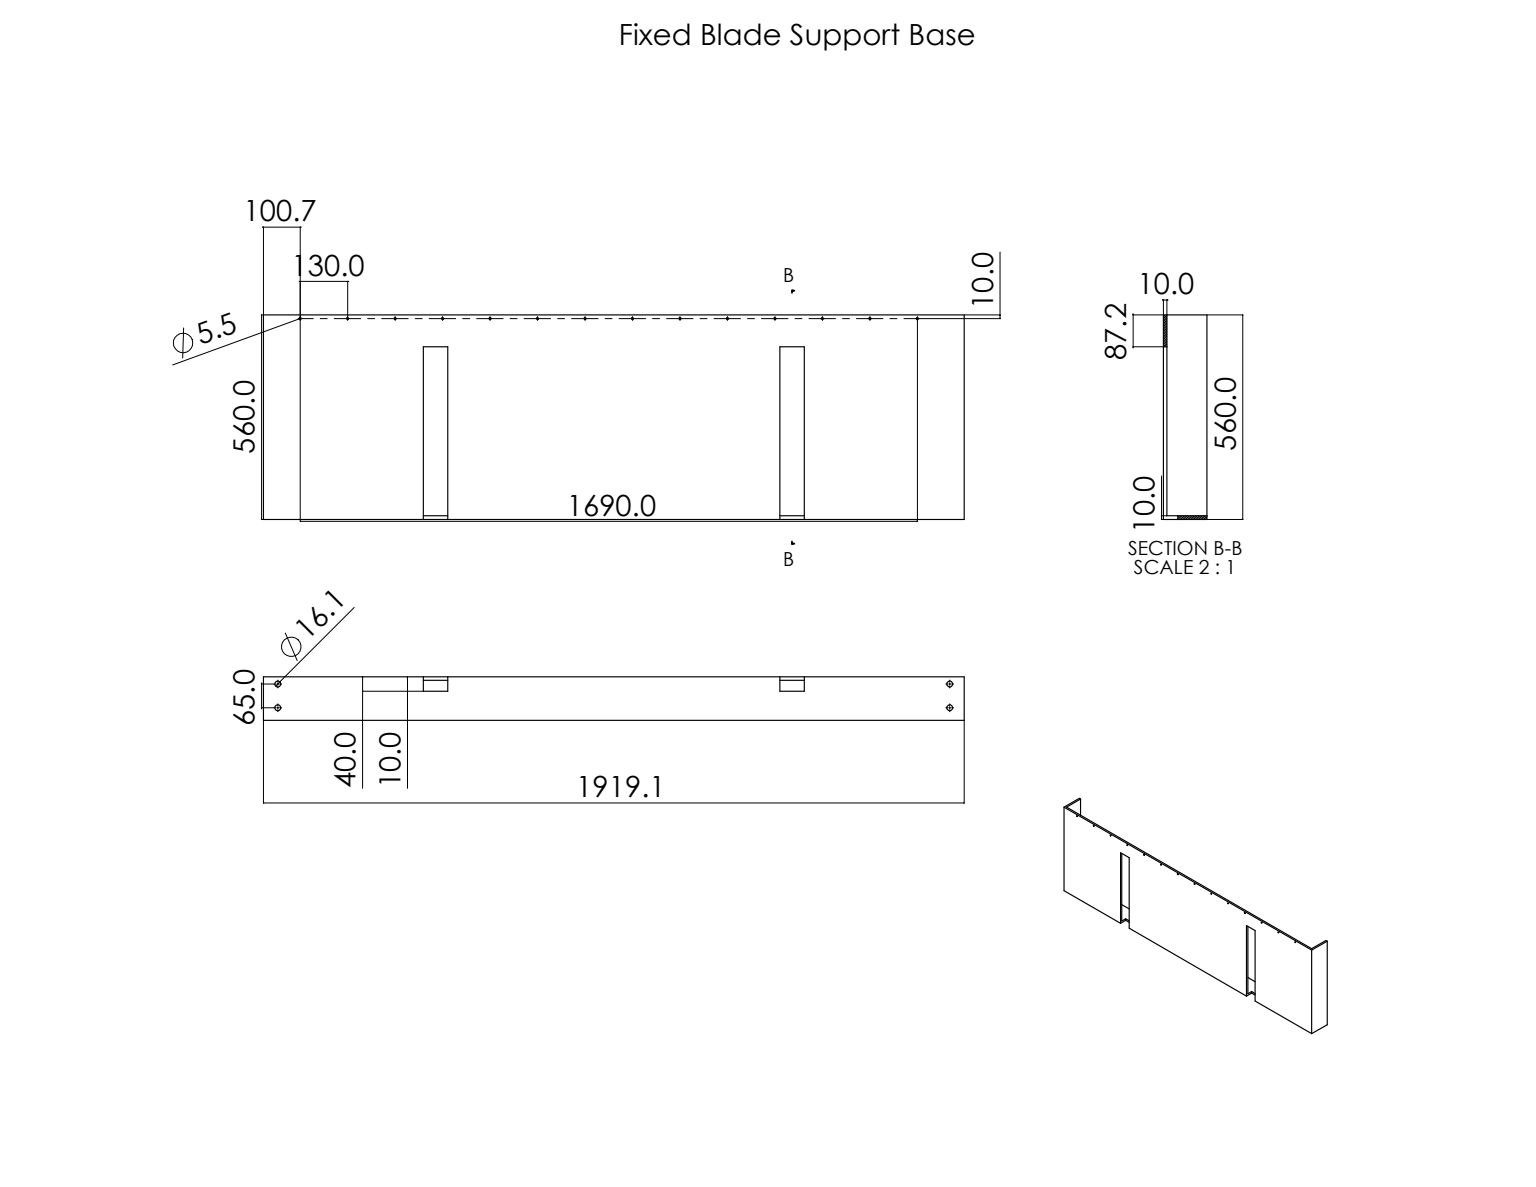
ISO-10303-21;
HEADER;
FILE_DESCRIPTION (('STEP AP214'),
    '1' );
FILE_NAME ('Fixed Blade Support Base.step',
    '2026-10-21T17:07:05',
    ( '' ),
    ( '' ),
    'SwSTEP 2.0',
    'SolidWorks 2025',
    '' );
FILE_SCHEMA (( 'AUTOMOTIVE_DESIGN' ));
ENDSEC;

DATA;
#38=ADVANCED_FACE ( 'NONE', ( #15558 ), #12093, .F. ) ;
#45=CARTESIAN_POINT ( 'NONE',  ( -454.7528517110260964, 240.0000000000001421, -122.7905160835438068 ) ) ;
#85=CARTESIAN_POINT ( 'NONE',  ( -949.5497976682736407, 240.0000000000002274, -2132.806278688367456 ) ) ;
#88=LINE ( 'NONE', #17428, #8305 ) ;
#95=DIRECTION ( 'NONE',  ( 1.000000000000000000, 0.000000000000000000, 0.000000000000000000 ) ) ;
#139=ORIENTED_EDGE ( 'NONE', *, *, #25849, .T. ) ;
#162=CARTESIAN_POINT ( 'NONE',  ( -208.8365100919714052, 260.0000000000001137, -197.2499999999928377 ) ) ;
#228=EDGE_LOOP ( 'NONE', ( #38649, #28007, #19169, #34955 ) ) ;
#282=VERTEX_POINT ( 'NONE', #6289 ) ;
#296=VERTEX_POINT ( 'NONE', #37011 ) ;
#303=CARTESIAN_POINT ( 'NONE',  ( -468.8365100919714337, 260.0000000000001705, -199.9999999999908766 ) ) ;
#305=ORIENTED_EDGE ( 'NONE', *, *, #27775, .T. ) ;
#308=DIRECTION ( 'NONE',  ( -1.880165489482579047E-16, -1.000000000000000000, -0.000000000000000000 ) ) ;
#338=VERTEX_POINT ( 'NONE', #40712 ) ;
#378=DIRECTION ( 'NONE',  ( -1.880165489482579047E-16, -1.000000000000000000, -0.000000000000000000 ) ) ;
#386=CIRCLE ( 'NONE', #29134, 2.749999999999919176 ) ;
#402=EDGE_CURVE ( 'NONE', #20839, #5125, #41180, .T. ) ;
#424=CARTESIAN_POINT ( 'NONE',  ( 454.7528517110262101, 239.9999999999999716, -122.7905160835442615 ) ) ;
#426=EDGE_CURVE ( 'NONE', #13538, #14856, #40502, .T. ) ;
#555=DIRECTION ( 'NONE',  ( -1.000000000000000000, 0.000000000000000000, 0.000000000000000000 ) ) ;
#590=ORIENTED_EDGE ( 'NONE', *, *, #29552, .T. ) ;
#593=VECTOR ( 'NONE', #7682, 1000.000000000000000 ) ;
#640=EDGE_CURVE ( 'NONE', #10075, #33702, #9985, .T. ) ;
#654=DIRECTION ( 'NONE',  ( -0.000000000000000000, 1.000000000000000000, -0.000000000000000000 ) ) ;
#709=ORIENTED_EDGE ( 'NONE', *, *, #5098, .T. ) ;
#718=ORIENTED_EDGE ( 'NONE', *, *, #22962, .T. ) ;
#728=EDGE_CURVE ( 'NONE', #13253, #15260, #21743, .T. ) ;
#739=CARTESIAN_POINT ( 'NONE',  ( 928.0249999999991815, 219.9999999999998863, 339.9999999999999432 ) ) ;
#767=ADVANCED_FACE ( 'NONE', ( #39786 ), #14838, .T. ) ;
#770=CARTESIAN_POINT ( 'NONE',  ( 919.9999999999993179, 154.9999999999998863, -360.0000000000000000 ) ) ;
#777=PLANE ( 'NONE',  #9882 ) ;
#791=VERTEX_POINT ( 'NONE', #739 ) ;
#796=CARTESIAN_POINT ( 'NONE',  ( -919.9999999999993179, 154.9999999999998863, 339.9999999999999432 ) ) ;
#804=ORIENTED_EDGE ( 'NONE', *, *, #1226, .T. ) ;
#824=CIRCLE ( 'NONE', #26615, 2.749999999999808153 ) ;
#853=( NAMED_UNIT ( * ) PLANE_ANGLE_UNIT ( ) SI_UNIT ( $, .RADIAN. ) );
#874=ORIENTED_EDGE ( 'NONE', *, *, #5250, .T. ) ;
#880=CARTESIAN_POINT ( 'NONE',  ( -728.8365100919714905, 260.0000000000001705, -197.2499999999891998 ) ) ;
#883=ORIENTED_EDGE ( 'NONE', *, *, #3255, .T. ) ;
#897=EDGE_LOOP ( 'NONE', ( #13761, #35388, #39807, #18362, #590, #6557 ) ) ;
#913=ADVANCED_FACE ( 'NONE', ( #39558 ), #7665, .T. ) ;
#925=CARTESIAN_POINT ( 'NONE',  ( 454.7528517110262101, 199.9999999999999432, -122.7905160835442615 ) ) ;
#928=VERTEX_POINT ( 'NONE', #4438 ) ;
#948=DIRECTION ( 'NONE',  ( -0.000000000000000000, 1.000000000000000000, -0.000000000000000000 ) ) ;
#955=EDGE_CURVE ( 'NONE', #16933, #23058, #18525, .T. ) ;
#977=ORIENTED_EDGE ( 'NONE', *, *, #34820, .T. ) ;
#990=CARTESIAN_POINT ( 'NONE',  ( -78.83651009197140525, 240.0000000000000853, -199.9999999999936051 ) ) ;
#999=CARTESIAN_POINT ( 'NONE',  ( -598.8365100919716042, 240.0000000000001705, -199.9999999999899671 ) ) ;
#1040=DIRECTION ( 'NONE',  ( -1.880165489482579047E-16, -1.000000000000000000, -0.000000000000000000 ) ) ;
#1042=ORIENTED_EDGE ( 'NONE', *, *, #30616, .F. ) ;
#1067=AXIS2_PLACEMENT_3D ( 'NONE', #33139, #27331, #40964 ) ;
#1084=AXIS2_PLACEMENT_3D ( 'NONE', #12147, #33380, #29263 ) ;
#1107=LINE ( 'NONE', #18453, #27055 ) ;
#1118=VECTOR ( 'NONE', #10969, 1000.000000000000000 ) ;
#1127=EDGE_LOOP ( 'NONE', ( #7257, #34123, #1263, #14595 ) ) ;
#1141=AXIS2_PLACEMENT_3D ( 'NONE', #10530, #3393, #38486 ) ;
#1148=AXIS2_PLACEMENT_3D ( 'NONE', #41013, #19989, #15837 ) ;
#1149=VECTOR ( 'NONE', #41633, 1000.000000000000000 ) ;
#1168=AXIS2_PLACEMENT_3D ( 'NONE', #303, #36103, #29173 ) ;
#1182=EDGE_CURVE ( 'NONE', #41190, #5430, #42343, .T. ) ;
#1199=EDGE_LOOP ( 'NONE', ( #16946, #35690 ) ) ;
#1226=EDGE_CURVE ( 'NONE', #32683, #45635, #5657, .T. ) ;
#1231=DIRECTION ( 'NONE',  ( 1.000000000000000000, 0.000000000000000000, 0.000000000000000000 ) ) ;
#1256=CARTESIAN_POINT ( 'NONE',  ( 919.9999999999993179, 219.9999999999998863, 339.9999999999999432 ) ) ;
#1263=ORIENTED_EDGE ( 'NONE', *, *, #19291, .T. ) ;
#1264=CARTESIAN_POINT ( 'NONE',  ( -208.8365100919714052, 240.0000000000001137, -199.9999999999926956 ) ) ;
#1270=AXIS2_PLACEMENT_3D ( 'NONE', #40692, #30517, #33770 ) ;
#1282=CARTESIAN_POINT ( 'NONE',  ( 521.6730038022808458, -9.808315785437627339E-14, 339.9999999999999432 ) ) ;
#1283=CARTESIAN_POINT ( 'NONE',  ( 454.7528517110261532, -8.550106180308601742E-14, 350.0000000000000000 ) ) ;
#1341=DIRECTION ( 'NONE',  ( -0.000000000000000000, 1.000000000000000000, -0.000000000000000000 ) ) ;
#1349=CARTESIAN_POINT ( 'NONE',  ( -521.6730038022808458, 230.0000000000001421, -122.7905160835438068 ) ) ;
#1382=VERTEX_POINT ( 'NONE', #27582 ) ;
#1385=CARTESIAN_POINT ( 'NONE',  ( -521.6730038022808458, 240.0000000000001705, -122.7905160835438068 ) ) ;
#1433=AXIS2_PLACEMENT_3D ( 'NONE', #27341, #16953, #45130 ) ;
#1438=CARTESIAN_POINT ( 'NONE',  ( 701.1634899080286232, 229.9999999999999147, -199.9999999999990337 ) ) ;
#1441=VERTEX_POINT ( 'NONE', #34968 ) ;
#1448=DIRECTION ( 'NONE',  ( -1.880165489482579047E-16, -1.000000000000000000, -0.000000000000000000 ) ) ;
#1468=UNCERTAINTY_MEASURE_WITH_UNIT (LENGTH_MEASURE( 1.000000000000000082E-05 ), #40729, 'distance_accuracy_value', 'NONE');
#1475=EDGE_CURVE ( 'NONE', #11526, #30518, #11359, .T. ) ;
#1533=EDGE_LOOP ( 'NONE', ( #21943, #37400, #33913, #3178 ) ) ;
#1581=EDGE_CURVE ( 'NONE', #44771, #12718, #29778, .T. ) ;
#1586=EDGE_LOOP ( 'NONE', ( #29834, #5171 ) ) ;
#1589=ADVANCED_FACE ( 'NONE', ( #18120 ), #7960, .F. ) ;
#1653=CARTESIAN_POINT ( 'NONE',  ( -858.8365100919713768, 240.0000000000002274, -197.2499999999882903 ) ) ;
#1658=CIRCLE ( 'NONE', #5350, 2.749999999999919176 ) ;
#1661=DIRECTION ( 'NONE',  ( 0.000000000000000000, 0.000000000000000000, 1.000000000000000000 ) ) ;
#1685=VERTEX_POINT ( 'NONE', #28739 ) ;
#1713=DIRECTION ( 'NONE',  ( 0.000000000000000000, 0.000000000000000000, 1.000000000000000000 ) ) ;
#1766=CYLINDRICAL_SURFACE ( 'NONE', #37801, 2.749999999999835687 ) ;
#1769=VERTEX_POINT ( 'NONE', #11404 ) ;
#1782=AXIS2_PLACEMENT_3D ( 'NONE', #9208, #19373, #33692 ) ;
#1802=EDGE_CURVE ( 'NONE', #5430, #41897, #11642, .T. ) ;
#1807=EDGE_CURVE ( 'NONE', #23028, #44488, #4925, .T. ) ;
#1818=AXIS2_PLACEMENT_3D ( 'NONE', #5730, #9193, #2253 ) ;
#1843=AXIS2_PLACEMENT_3D ( 'NONE', #23538, #17085, #9694 ) ;
#1872=EDGE_LOOP ( 'NONE', ( #17747, #14797 ) ) ;
#1891=CYLINDRICAL_SURFACE ( 'NONE', #26649, 2.749999999999863665 ) ;
#1902=FACE_BOUND ( 'NONE', #43260, .T. ) ;
#2009=PLANE ( 'NONE',  #5339 ) ;
#2099=VERTEX_POINT ( 'NONE', #40706 ) ;
#2160=EDGE_CURVE ( 'NONE', #33957, #338, #42375, .T. ) ;
#2235=CARTESIAN_POINT ( 'NONE',  ( 311.1634899080286232, 229.9999999999999716, -199.9999999999963336 ) ) ;
#2245=PRODUCT ( 'Fixed Blade Support Base', 'Fixed Blade Support Base', '', ( #30746 ) ) ;
#2253=DIRECTION ( 'NONE',  ( 1.000000000000000000, 0.000000000000000000, 0.000000000000000000 ) ) ;
#2263=DIRECTION ( 'NONE',  ( -1.880165489482579047E-16, -1.000000000000000000, -0.000000000000000000 ) ) ;
#2300=DIRECTION ( 'NONE',  ( 1.000000000000000000, 0.000000000000000000, 0.000000000000000000 ) ) ;
#2334=DIRECTION ( 'NONE',  ( 1.000000000000000000, -1.880165489482579047E-16, -0.000000000000000000 ) ) ;
#2362=CYLINDRICAL_SURFACE ( 'NONE', #32139, 2.749999999999863665 ) ;
#2393=DIRECTION ( 'NONE',  ( 0.000000000000000000, 0.000000000000000000, 1.000000000000000000 ) ) ;
#2412=CARTESIAN_POINT ( 'NONE',  ( -728.8365100919714905, 230.0000000000001705, -199.9999999999890861 ) ) ;
#2464=CARTESIAN_POINT ( 'NONE',  ( 571.1634899080285095, 259.9999999999999432, -197.2499999999982947 ) ) ;
#2466=ORIENTED_EDGE ( 'NONE', *, *, #29751, .T. ) ;
#2476=ORIENTED_EDGE ( 'NONE', *, *, #21855, .F. ) ;
#2503=AXIS2_PLACEMENT_3D ( 'NONE', #20702, #6847, #3401 ) ;
#2540=AXIS2_PLACEMENT_3D ( 'NONE', #20368, #24281, #24744 ) ;
#2545=EDGE_LOOP ( 'NONE', ( #19262, #7741, #30157, #11975 ) ) ;
#2557=AXIS2_PLACEMENT_3D ( 'NONE', #30153, #39499, #12154 ) ;
#2612=ORIENTED_EDGE ( 'NONE', *, *, #26636, .F. ) ;
#2616=DIRECTION ( 'NONE',  ( 0.000000000000000000, 0.000000000000000000, 1.000000000000000000 ) ) ;
#2632=ORIENTED_EDGE ( 'NONE', *, *, #41103, .T. ) ;
#2675=CARTESIAN_POINT ( 'NONE',  ( -454.7528517110260964, 240.0000000000001421, -122.7905160835438068 ) ) ;
#2710=ORIENTED_EDGE ( 'NONE', *, *, #30034, .T. ) ;
#2762=ORIENTED_EDGE ( 'NONE', *, *, #25210, .F. ) ;
#2775=CARTESIAN_POINT ( 'NONE',  ( -911.9749999999993406, 154.9999999999998863, -360.0000000000000000 ) ) ;
#2811=CARTESIAN_POINT ( 'NONE',  ( 51.16348990802859475, 230.0000000000000284, -197.2499999999946851 ) ) ;
#2837=DIRECTION ( 'NONE',  ( 0.000000000000000000, 0.000000000000000000, 1.000000000000000000 ) ) ;
#2846=DIRECTION ( 'NONE',  ( 0.000000000000000000, 0.000000000000000000, 1.000000000000000000 ) ) ;
#2882=DIRECTION ( 'NONE',  ( -0.000000000000000000, 1.000000000000000000, -0.000000000000000000 ) ) ;
#2940=CARTESIAN_POINT ( 'NONE',  ( 959.5497976682736407, 120.6654763175833693, -209.9999999999999716 ) ) ;
#2977=EDGE_LOOP ( 'NONE', ( #34128, #28219, #43060, #8539 ) ) ;
#3069=EDGE_LOOP ( 'NONE', ( #41787, #15073, #40615, #43520 ) ) ;
#3119=CIRCLE ( 'NONE', #40733, 2.749999999999863665 ) ;
#3178=ORIENTED_EDGE ( 'NONE', *, *, #9445, .F. ) ;
#3198=LINE ( 'NONE', #20529, #22575 ) ;
#3208=VECTOR ( 'NONE', #4412, 1000.000000000000000 ) ;
#3241=DIRECTION ( 'NONE',  ( 1.880165489482579047E-16, 1.000000000000000000, 0.000000000000000000 ) ) ;
#3255=EDGE_CURVE ( 'NONE', #5332, #39962, #34406, .T. ) ;
#3261=ORIENTED_EDGE ( 'NONE', *, *, #14766, .F. ) ;
#3301=FACE_OUTER_BOUND ( 'NONE', #15485, .T. ) ;
#3304=EDGE_LOOP ( 'NONE', ( #13111, #25405, #11101, #40410 ) ) ;
#3350=AXIS2_PLACEMENT_3D ( 'NONE', #35593, #3969, #7913 ) ;
#3392=CYLINDRICAL_SURFACE ( 'NONE', #42536, 2.749999999999835687 ) ;
#3393=DIRECTION ( 'NONE',  ( -0.000000000000000000, 1.000000000000000000, -0.000000000000000000 ) ) ;
#3397=DIRECTION ( 'NONE',  ( 1.000000000000000000, 0.000000000000000000, 0.000000000000000000 ) ) ;
#3401=DIRECTION ( 'NONE',  ( -1.000000000000000000, 0.000000000000000000, 0.000000000000000000 ) ) ;
#3427=VERTEX_POINT ( 'NONE', #29080 ) ;
#3447=EDGE_LOOP ( 'NONE', ( #7412, #17344 ) ) ;
#3452=DIRECTION ( 'NONE',  ( -0.000000000000000000, -0.000000000000000000, 1.000000000000000000 ) ) ;
#3455=VECTOR ( 'NONE', #31937, 1000.000000000000000 ) ;
#3458=AXIS2_PLACEMENT_3D ( 'NONE', #40138, #18451, #11058 ) ;
#3495=AXIS2_PLACEMENT_3D ( 'NONE', #13303, #23897, #38017 ) ;
#3503=ORIENTED_EDGE ( 'NONE', *, *, #13757, .T. ) ;
#3519=DIRECTION ( 'NONE',  ( 1.000000000000000000, 0.000000000000000000, 0.000000000000000000 ) ) ;
#3556=EDGE_LOOP ( 'NONE', ( #5524, #38328, #27108, #43854 ) ) ;
#3591=EDGE_CURVE ( 'NONE', #43844, #27381, #39729, .T. ) ;
#3630=DIRECTION ( 'NONE',  ( -0.000000000000000000, -0.000000000000000000, 1.000000000000000000 ) ) ;
#3650=ORIENTED_EDGE ( 'NONE', *, *, #36433, .F. ) ;
#3678=CARTESIAN_POINT ( 'NONE',  ( 521.6730038022808458, 199.9999999999999147, 350.0000000000000000 ) ) ;
#3695=FACE_BOUND ( 'NONE', #34718, .T. ) ;
#3710=DIRECTION ( 'NONE',  ( 1.000000000000000000, 0.000000000000000000, 0.000000000000000000 ) ) ;
#3770=ORIENTED_EDGE ( 'NONE', *, *, #22696, .F. ) ;
#3835=EDGE_LOOP ( 'NONE', ( #2476, #20852, #37122, #36881 ) ) ;
#3840=CYLINDRICAL_SURFACE ( 'NONE', #29331, 2.749999999999863665 ) ;
#3889=CARTESIAN_POINT ( 'NONE',  ( 949.5497976682736407, 229.9999999999998579, -210.0000000000000000 ) ) ;
#3943=CARTESIAN_POINT ( 'NONE',  ( 311.1634899080286232, 229.9999999999999716, -202.7499999999961915 ) ) ;
#3945=DIRECTION ( 'NONE',  ( -1.880165489482579047E-16, -1.000000000000000000, 0.000000000000000000 ) ) ;
#3957=DIRECTION ( 'NONE',  ( 1.000000000000000000, 0.000000000000000000, 0.000000000000000000 ) ) ;
#3969=DIRECTION ( 'NONE',  ( 4.147566128926363633E-16, 1.000000000000000000, -0.000000000000000000 ) ) ;
#4034=DIRECTION ( 'NONE',  ( -0.000000000000000000, -0.000000000000000000, 1.000000000000000000 ) ) ;
#4072=DIRECTION ( 'NONE',  ( -0.000000000000000000, 1.000000000000000000, -0.000000000000000000 ) ) ;
#4094=DIRECTION ( 'NONE',  ( 1.000000000000000000, -4.147566128926363633E-16, 0.000000000000000000 ) ) ;
#4099=AXIS2_PLACEMENT_3D ( 'NONE', #15118, #4034, #17897 ) ;
#4101=CARTESIAN_POINT ( 'NONE',  ( -598.8365100919716042, 230.0000000000001421, -199.9999999999899671 ) ) ;
#4111=EDGE_CURVE ( 'NONE', #1382, #39820, #21040, .T. ) ;
#4156=VECTOR ( 'NONE', #20629, 1000.000000000000000 ) ;
#4228=AXIS2_PLACEMENT_3D ( 'NONE', #19562, #44748, #44506 ) ;
#4250=DIRECTION ( 'NONE',  ( -0.000000000000000000, -0.000000000000000000, 1.000000000000000000 ) ) ;
#4263=DIRECTION ( 'NONE',  ( -1.880165489482579047E-16, -1.000000000000000000, -0.000000000000000000 ) ) ;
#4290=EDGE_LOOP ( 'NONE', ( #8058, #41150 ) ) ;
#4307=DIRECTION ( 'NONE',  ( -1.880165489482579047E-16, -1.000000000000000000, 0.000000000000000000 ) ) ;
#4314=CARTESIAN_POINT ( 'NONE',  ( 441.1634899080286232, 240.0000000000000000, -197.2499999999973852 ) ) ;
#4343=ORIENTED_EDGE ( 'NONE', *, *, #8870, .T. ) ;
#4355=FACE_BOUND ( 'NONE', #4290, .T. ) ;
#4357=CARTESIAN_POINT ( 'NONE',  ( -858.8365100919713768, 240.0000000000002274, -199.9999999999881481 ) ) ;
#4374=EDGE_CURVE ( 'NONE', #28460, #35455, #44677, .T. ) ;
#4408=ORIENTED_EDGE ( 'NONE', *, *, #39387, .F. ) ;
#4412=DIRECTION ( 'NONE',  ( 0.000000000000000000, 0.000000000000000000, 1.000000000000000000 ) ) ;
#4417=EDGE_CURVE ( 'NONE', #5332, #27330, #8529, .T. ) ;
#4438=CARTESIAN_POINT ( 'NONE',  ( 911.9749999999993406, 219.9999999999998863, 350.0000000000000000 ) ) ;
#4493=DIRECTION ( 'NONE',  ( -1.880165489482579047E-16, -1.000000000000000000, -0.000000000000000000 ) ) ;
#4501=DIRECTION ( 'NONE',  ( -0.000000000000000000, -0.000000000000000000, -1.000000000000000000 ) ) ;
#4503=ORIENTED_EDGE ( 'NONE', *, *, #34012, .T. ) ;
#4515=CARTESIAN_POINT ( 'NONE',  ( 51.16348990802859475, 230.0000000000000284, -199.9999999999945146 ) ) ;
#4523=CYLINDRICAL_SURFACE ( 'NONE', #21937, 2.749999999999835687 ) ;
#4528=PLANE ( 'NONE',  #30383 ) ;
#4587=CARTESIAN_POINT ( 'NONE',  ( -959.5497976682736407, 120.6654763175833693, 350.0000000000000000 ) ) ;
#4615=ORIENTED_EDGE ( 'NONE', *, *, #44639, .T. ) ;
#4617=EDGE_LOOP ( 'NONE', ( #37789, #37136, #11659, #3650 ) ) ;
#4645=EDGE_CURVE ( 'NONE', #13769, #7179, #33603, .T. ) ;
#4682=FACE_BOUND ( 'NONE', #31928, .T. ) ;
#4693=LINE ( 'NONE', #17881, #18176 ) ;
#4697=CIRCLE ( 'NONE', #30499, 2.749999999999863665 ) ;
#4724=ORIENTED_EDGE ( 'NONE', *, *, #38163, .F. ) ;
#4754=CARTESIAN_POINT ( 'NONE',  ( 51.16348990802859475, 240.0000000000000568, -199.9999999999945146 ) ) ;
#4780=AXIS2_PLACEMENT_3D ( 'NONE', #5364, #25726, #15110 ) ;
#4795=FACE_BOUND ( 'NONE', #34607, .T. ) ;
#4812=CIRCLE ( 'NONE', #1148, 8.024999999999948841 ) ;
#4841=CIRCLE ( 'NONE', #29926, 2.749999999999919176 ) ;
#4861=CIRCLE ( 'NONE', #30681, 8.024999999999948841 ) ;
#4901=ORIENTED_EDGE ( 'NONE', *, *, #1802, .F. ) ;
#4911=VECTOR ( 'NONE', #29518, 1000.000000000000000 ) ;
#4925=LINE ( 'NONE', #22028, #32023 ) ;
#4927=EDGE_CURVE ( 'NONE', #44845, #9329, #18884, .T. ) ;
#4933=CYLINDRICAL_SURFACE ( 'NONE', #4780, 2.749999999999863665 ) ;
#4939=AXIS2_PLACEMENT_3D ( 'NONE', #43926, #18779, #15992 ) ;
#4974=CIRCLE ( 'NONE', #12362, 8.024999999999948841 ) ;
#5098=EDGE_CURVE ( 'NONE', #12788, #16603, #29845, .T. ) ;
#5125=VERTEX_POINT ( 'NONE', #15541 ) ;
#5129=CIRCLE ( 'NONE', #1433, 2.749999999999835687 ) ;
#5139=EDGE_CURVE ( 'NONE', #34173, #10227, #7948, .T. ) ;
#5156=CARTESIAN_POINT ( 'NONE',  ( 959.5497976682736407, 239.9999999999998863, -2132.806278688367456 ) ) ;
#5160=DIRECTION ( 'NONE',  ( 1.000000000000000000, 0.000000000000000000, 0.000000000000000000 ) ) ;
#5171=ORIENTED_EDGE ( 'NONE', *, *, #43893, .T. ) ;
#5229=EDGE_LOOP ( 'NONE', ( #15133, #26425 ) ) ;
#5239=EDGE_CURVE ( 'NONE', #43290, #42970, #27072, .T. ) ;
#5249=CARTESIAN_POINT ( 'NONE',  ( 959.5497976682736407, 120.6654763175833693, -2132.806278688367456 ) ) ;
#5250=EDGE_CURVE ( 'NONE', #20839, #5289, #39638, .T. ) ;
#5289=VERTEX_POINT ( 'NONE', #30288 ) ;
#5332=VERTEX_POINT ( 'NONE', #40482 ) ;
#5339=AXIS2_PLACEMENT_3D ( 'NONE', #5930, #26716, #13330 ) ;
#5348=ORIENTED_EDGE ( 'NONE', *, *, #1226, .F. ) ;
#5350=AXIS2_PLACEMENT_3D ( 'NONE', #8388, #11398, #25483 ) ;
#5354=CARTESIAN_POINT ( 'NONE',  ( 831.1634899080286232, 229.9999999999998863, -197.2500000000000853 ) ) ;
#5364=CARTESIAN_POINT ( 'NONE',  ( 701.1634899080286232, 259.9999999999999432, -199.9999999999990337 ) ) ;
#5367=CIRCLE ( 'NONE', #26007, 2.749999999999863665 ) ;
#5371=DIRECTION ( 'NONE',  ( 0.000000000000000000, 0.000000000000000000, 1.000000000000000000 ) ) ;
#5384=CARTESIAN_POINT ( 'NONE',  ( 454.7528517110262101, 239.9999999999999716, -122.7905160835442615 ) ) ;
#5397=CARTESIAN_POINT ( 'NONE',  ( -919.9999999999993179, 154.9999999999998863, 350.0000000000000000 ) ) ;
#5414=DIRECTION ( 'NONE',  ( -1.880165489482579047E-16, -1.000000000000000000, -0.000000000000000000 ) ) ;
#5430=VERTEX_POINT ( 'NONE', #12737 ) ;
#5433=AXIS2_PLACEMENT_3D ( 'NONE', #22081, #32258, #21856 ) ;
#5446=ORIENTED_EDGE ( 'NONE', *, *, #32624, .F. ) ;
#5492=CARTESIAN_POINT ( 'NONE',  ( 311.1634899080286232, 240.0000000000000000, -202.7499999999961915 ) ) ;
#5496=ORIENTED_EDGE ( 'NONE', *, *, #20182, .F. ) ;
#5499=EDGE_CURVE ( 'NONE', #14856, #20856, #39484, .T. ) ;
#5503=EDGE_LOOP ( 'NONE', ( #40837, #6028 ) ) ;
#5506=VECTOR ( 'NONE', #5595, 1000.000000000000000 ) ;
#5522=VECTOR ( 'NONE', #4307, 1000.000000000000000 ) ;
#5524=ORIENTED_EDGE ( 'NONE', *, *, #32500, .T. ) ;
#5541=EDGE_CURVE ( 'NONE', #6874, #9331, #11602, .T. ) ;
#5585=ORIENTED_EDGE ( 'NONE', *, *, #17111, .F. ) ;
#5591=DIRECTION ( 'NONE',  ( -0.000000000000000000, 1.000000000000000000, -0.000000000000000000 ) ) ;
#5595=DIRECTION ( 'NONE',  ( 1.000000000000000000, -1.880165489482579047E-16, -0.000000000000000000 ) ) ;
#5626=ORIENTED_EDGE ( 'NONE', *, *, #14615, .F. ) ;
#5635=FACE_BOUND ( 'NONE', #29931, .T. ) ;
#5638=CARTESIAN_POINT ( 'NONE',  ( -949.5497976682736407, 120.6654763175833693, -2132.806278688367456 ) ) ;
#5657=LINE ( 'NONE', #34278, #45285 ) ;
#5679=DIRECTION ( 'NONE',  ( -0.000000000000000000, 1.000000000000000000, -0.000000000000000000 ) ) ;
#5694=ORIENTED_EDGE ( 'NONE', *, *, #44442, .T. ) ;
#5710=LINE ( 'NONE', #23474, #20423 ) ;
#5717=DIRECTION ( 'NONE',  ( 1.000000000000000000, 0.000000000000000000, 0.000000000000000000 ) ) ;
#5730=CARTESIAN_POINT ( 'NONE',  ( 919.9999999999993179, 219.9999999999998863, -360.0000000000000000 ) ) ;
#5760=LINE ( 'NONE', #33929, #19426 ) ;
#5802=ORIENTED_EDGE ( 'NONE', *, *, #33989, .F. ) ;
#5810=VERTEX_POINT ( 'NONE', #1349 ) ;
#5814=ADVANCED_FACE ( 'NONE', ( #19974 ), #36448, .T. ) ;
#5820=LINE ( 'NONE', #16902, #44029 ) ;
#5848=VERTEX_POINT ( 'NONE', #15229 ) ;
#5869=FACE_OUTER_BOUND ( 'NONE', #22229, .T. ) ;
#5870=ORIENTED_EDGE ( 'NONE', *, *, #15575, .F. ) ;
#5906=CARTESIAN_POINT ( 'NONE',  ( -911.9749999999993406, 219.9999999999998863, 339.9999999999999432 ) ) ;
#5930=CARTESIAN_POINT ( 'NONE',  ( 454.7528517110262101, 199.9999999999999432, -122.7905160835442615 ) ) ;
#5955=VERTEX_POINT ( 'NONE', #4587 ) ;
#5978=VERTEX_POINT ( 'NONE', #9357 ) ;
#6013=AXIS2_PLACEMENT_3D ( 'NONE', #18296, #15281, #3957 ) ;
#6028=ORIENTED_EDGE ( 'NONE', *, *, #5250, .F. ) ;
#6075=DIRECTION ( 'NONE',  ( 1.000000000000000000, 0.000000000000000000, 0.000000000000000000 ) ) ;
#6093=ORIENTED_EDGE ( 'NONE', *, *, #29552, .F. ) ;
#6158=DIRECTION ( 'NONE',  ( 1.000000000000000000, 0.000000000000000000, 0.000000000000000000 ) ) ;
#6177=FACE_BOUND ( 'NONE', #14391, .T. ) ;
#6189=EDGE_LOOP ( 'NONE', ( #30273, #41536 ) ) ;
#6220=DIRECTION ( 'NONE',  ( -0.000000000000000000, 1.000000000000000000, -0.000000000000000000 ) ) ;
#6225=CARTESIAN_POINT ( 'NONE',  ( 959.5497976682736407, 120.6654763175833693, -209.9999999999999716 ) ) ;
#6264=CARTESIAN_POINT ( 'NONE',  ( -911.9749999999993406, 154.9999999999998863, 350.0000000000000000 ) ) ;
#6289=CARTESIAN_POINT ( 'NONE',  ( 928.0249999999991815, 219.9999999999998863, 350.0000000000000000 ) ) ;
#6316=ORIENTED_EDGE ( 'NONE', *, *, #42173, .T. ) ;
#6322=DIRECTION ( 'NONE',  ( -0.000000000000000000, 1.000000000000000000, -0.000000000000000000 ) ) ;
#6330=CARTESIAN_POINT ( 'NONE',  ( 8.295132257852724189E-14, 199.9999999999999147, 339.9999999999999432 ) ) ;
#6347=FACE_OUTER_BOUND ( 'NONE', #897, .T. ) ;
#6375=ORIENTED_EDGE ( 'NONE', *, *, #17668, .T. ) ;
#6412=CYLINDRICAL_SURFACE ( 'NONE', #42927, 8.024999999999948841 ) ;
#6422=DIRECTION ( 'NONE',  ( 0.000000000000000000, 0.000000000000000000, 1.000000000000000000 ) ) ;
#6431=ORIENTED_EDGE ( 'NONE', *, *, #23149, .F. ) ;
#6432=AXIS2_PLACEMENT_3D ( 'NONE', #1438, #19440, #12304 ) ;
#6437=ORIENTED_EDGE ( 'NONE', *, *, #22489, .T. ) ;
#6521=DIRECTION ( 'NONE',  ( -0.000000000000000000, -0.000000000000000000, -1.000000000000000000 ) ) ;
#6552=LINE ( 'NONE', #27801, #12513 ) ;
#6557=ORIENTED_EDGE ( 'NONE', *, *, #10256, .F. ) ;
#6628=PLANE ( 'NONE',  #2503 ) ;
#6702=UNCERTAINTY_MEASURE_WITH_UNIT (LENGTH_MEASURE( 1.000000000000000082E-05 ), #15190, 'distance_accuracy_value', 'NONE');
#6715=CIRCLE ( 'NONE', #18541, 2.749999999999919176 ) ;
#6762=DIRECTION ( 'NONE',  ( -0.000000000000000000, 1.000000000000000000, -0.000000000000000000 ) ) ;
#6811=VECTOR ( 'NONE', #40991, 1000.000000000000000 ) ;
#6823=ORIENTED_EDGE ( 'NONE', *, *, #43817, .F. ) ;
#6847=DIRECTION ( 'NONE',  ( 0.000000000000000000, 0.000000000000000000, -1.000000000000000000 ) ) ;
#6865=CARTESIAN_POINT ( 'NONE',  ( -454.7528517110260964, 230.0000000000002274, 339.9999999999999432 ) ) ;
#6873=EDGE_CURVE ( 'NONE', #2099, #5978, #4693, .T. ) ;
#6874=VERTEX_POINT ( 'NONE', #21793 ) ;
#6887=CARTESIAN_POINT ( 'NONE',  ( -858.8365100919713768, 260.0000000000002274, -197.2499999999882903 ) ) ;
#6916=CARTESIAN_POINT ( 'NONE',  ( 831.1634899080286232, 229.9999999999998863, -199.9999999999999432 ) ) ;
#6919=EDGE_CURVE ( 'NONE', #20856, #7346, #12316, .T. ) ;
#6965=VECTOR ( 'NONE', #8165, 1000.000000000000000 ) ;
#7005=ORIENTED_EDGE ( 'NONE', *, *, #12262, .F. ) ;
#7007=EDGE_LOOP ( 'NONE', ( #41414, #44382, #26150, #19772 ) ) ;
#7090=FACE_OUTER_BOUND ( 'NONE', #2977, .T. ) ;
#7143=EDGE_CURVE ( 'NONE', #33570, #39336, #43847, .T. ) ;
#7179=VERTEX_POINT ( 'NONE', #43708 ) ;
#7200=ORIENTED_EDGE ( 'NONE', *, *, #39132, .F. ) ;
#7230=DIRECTION ( 'NONE',  ( 1.000000000000000000, 0.000000000000000000, 0.000000000000000000 ) ) ;
#7257=ORIENTED_EDGE ( 'NONE', *, *, #34820, .F. ) ;
#7293=DIRECTION ( 'NONE',  ( -0.000000000000000000, -0.000000000000000000, -1.000000000000000000 ) ) ;
#7327=CARTESIAN_POINT ( 'NONE',  ( -598.8365100919716042, 230.0000000000001421, -202.7499999999898250 ) ) ;
#7346=VERTEX_POINT ( 'NONE', #19686 ) ;
#7350=ORIENTED_EDGE ( 'NONE', *, *, #16570, .F. ) ;
#7412=ORIENTED_EDGE ( 'NONE', *, *, #28627, .T. ) ;
#7420=EDGE_CURVE ( 'NONE', #5430, #41190, #386, .T. ) ;
#7477=PRODUCT_DEFINITION_SHAPE ( 'NONE', 'NONE',  #39755 ) ;
#7510=EDGE_CURVE ( 'NONE', #3427, #33397, #40218, .T. ) ;
#7516=ORIENTED_EDGE ( 'NONE', *, *, #1182, .T. ) ;
#7538=FACE_OUTER_BOUND ( 'NONE', #9091, .T. ) ;
#7573=AXIS2_PLACEMENT_3D ( 'NONE', #34573, #37575, #33658 ) ;
#7590=LINE ( 'NONE', #26493, #27788 ) ;
#7661=DIRECTION ( 'NONE',  ( -0.000000000000000000, 1.000000000000000000, -0.000000000000000000 ) ) ;
#7665=PLANE ( 'NONE',  #3350 ) ;
#7682=DIRECTION ( 'NONE',  ( -0.000000000000000000, 1.000000000000000000, -0.000000000000000000 ) ) ;
#7715=DIRECTION ( 'NONE',  ( -0.000000000000000000, 1.000000000000000000, -0.000000000000000000 ) ) ;
#7741=ORIENTED_EDGE ( 'NONE', *, *, #37087, .T. ) ;
#7760=EDGE_LOOP ( 'NONE', ( #40509, #37942, #883, #18815 ) ) ;
#7811=VERTEX_POINT ( 'NONE', #8128 ) ;
#7888=CIRCLE ( 'NONE', #21885, 2.749999999999835687 ) ;
#7889=PLANE ( 'NONE',  #15988 ) ;
#7898=VECTOR ( 'NONE', #14870, 1000.000000000000000 ) ;
#7913=DIRECTION ( 'NONE',  ( -1.000000000000000000, 4.147566128926363633E-16, 0.000000000000000000 ) ) ;
#7948=LINE ( 'NONE', #25918, #11389 ) ;
#7960=CYLINDRICAL_SURFACE ( 'NONE', #12086, 2.749999999999863665 ) ;
#7967=FACE_BOUND ( 'NONE', #5503, .T. ) ;
#7973=CYLINDRICAL_SURFACE ( 'NONE', #4099, 8.024999999999948841 ) ;
#8008=LINE ( 'NONE', #12366, #5522 ) ;
#8013=FACE_OUTER_BOUND ( 'NONE', #10547, .T. ) ;
#8054=CYLINDRICAL_SURFACE ( 'NONE', #11775, 2.749999999999863665 ) ;
#8058=ORIENTED_EDGE ( 'NONE', *, *, #16308, .T. ) ;
#8077=CARTESIAN_POINT ( 'NONE',  ( 454.7528517110262101, 239.9999999999999716, -122.7905160835442615 ) ) ;
#8086=EDGE_CURVE ( 'NONE', #10075, #27381, #16168, .T. ) ;
#8116=VERTEX_POINT ( 'NONE', #24230 ) ;
#8122=CARTESIAN_POINT ( 'NONE',  ( 441.1634899080286232, 259.9999999999999432, -197.2499999999973852 ) ) ;
#8128=CARTESIAN_POINT ( 'NONE',  ( 454.7528517110262101, 230.0000000000002274, 339.9999999999999432 ) ) ;
#8151=EDGE_LOOP ( 'NONE', ( #43349, #34026, #29103, #8255 ) ) ;
#8165=DIRECTION ( 'NONE',  ( -0.000000000000000000, -0.000000000000000000, 1.000000000000000000 ) ) ;
#8169=CARTESIAN_POINT ( 'NONE',  ( 441.1634899080286232, 229.9999999999999716, -199.9999999999972431 ) ) ;
#8175=CARTESIAN_POINT ( 'NONE',  ( -728.8365100919714905, 260.0000000000001705, -202.7499999999889440 ) ) ;
#8181=FACE_BOUND ( 'NONE', #37850, .T. ) ;
#8216=CARTESIAN_POINT ( 'NONE',  ( 928.0249999999991815, 154.9999999999998863, -360.0000000000000000 ) ) ;
#8252=EDGE_CURVE ( 'NONE', #8116, #21264, #13620, .T. ) ;
#8255=ORIENTED_EDGE ( 'NONE', *, *, #45596, .F. ) ;
#8298=EDGE_CURVE ( 'NONE', #21010, #41897, #21777, .T. ) ;
#8305=VECTOR ( 'NONE', #31507, 1000.000000000000000 ) ;
#8322=FACE_OUTER_BOUND ( 'NONE', #3835, .T. ) ;
#8337=EDGE_CURVE ( 'NONE', #17262, #7179, #30947, .T. ) ;
#8388=CARTESIAN_POINT ( 'NONE',  ( -858.8365100919713768, 230.0000000000001990, -199.9999999999881481 ) ) ;
#8401=DIRECTION ( 'NONE',  ( 1.000000000000000000, -1.880165489482579047E-16, 0.000000000000000000 ) ) ;
#8424=ORIENTED_EDGE ( 'NONE', *, *, #20739, .T. ) ;
#8425=AXIS2_PLACEMENT_3D ( 'NONE', #1264, #11884, #22492 ) ;
#8427=VECTOR ( 'NONE', #39142, 1000.000000000000000 ) ;
#8497=EDGE_CURVE ( 'NONE', #5810, #24407, #30400, .T. ) ;
#8506=DIRECTION ( 'NONE',  ( 0.000000000000000000, 0.000000000000000000, 1.000000000000000000 ) ) ;
#8513=AXIS2_PLACEMENT_3D ( 'NONE', #33182, #37310, #23440 ) ;
#8524=CYLINDRICAL_SURFACE ( 'NONE', #24641, 2.749999999999863665 ) ;
#8529=CIRCLE ( 'NONE', #38040, 8.024999999999948841 ) ;
#8531=CARTESIAN_POINT ( 'NONE',  ( 454.7528517110261532, -8.550106180308601742E-14, 339.9999999999999432 ) ) ;
#8539=ORIENTED_EDGE ( 'NONE', *, *, #35945, .T. ) ;
#8570=DIRECTION ( 'NONE',  ( -1.880165489482579047E-16, -1.000000000000000000, -0.000000000000000000 ) ) ;
#8627=DIRECTION ( 'NONE',  ( -1.880165489482579047E-16, -1.000000000000000000, -0.000000000000000000 ) ) ;
#8638=FACE_BOUND ( 'NONE', #21534, .T. ) ;
#8678=CIRCLE ( 'NONE', #24148, 2.749999999999863665 ) ;
#8684=LINE ( 'NONE', #26884, #6811 ) ;
#8756=DIRECTION ( 'NONE',  ( 1.000000000000000000, -4.147566128926370535E-16, 0.000000000000000000 ) ) ;
#8759=ORIENTED_EDGE ( 'NONE', *, *, #41330, .T. ) ;
#8781=CARTESIAN_POINT ( 'NONE',  ( 701.1634899080286232, 239.9999999999999432, -202.7499999999988916 ) ) ;
#8833=PLANE ( 'NONE',  #4939 ) ;
#8840=DIRECTION ( 'NONE',  ( 1.000000000000000000, 0.000000000000000000, 0.000000000000000000 ) ) ;
#8852=CARTESIAN_POINT ( 'NONE',  ( 959.5497976682736407, 229.9999999999998579, -2132.806278688367456 ) ) ;
#8870=EDGE_CURVE ( 'NONE', #1685, #6874, #37338, .T. ) ;
#8977=ORIENTED_EDGE ( 'NONE', *, *, #34012, .F. ) ;
#8978=EDGE_LOOP ( 'NONE', ( #30270, #26130, #5585, #32312 ) ) ;
#9004=CARTESIAN_POINT ( 'NONE',  ( -208.8365100919714052, 230.0000000000000853, -199.9999999999926956 ) ) ;
#9015=CIRCLE ( 'NONE', #9744, 2.749999999999835687 ) ;
#9083=ORIENTED_EDGE ( 'NONE', *, *, #39102, .T. ) ;
#9091=EDGE_LOOP ( 'NONE', ( #35921, #977, #29837, #29456 ) ) ;
#9179=ADVANCED_FACE ( 'NONE', ( #45656 ), #14006, .F. ) ;
#9193=DIRECTION ( 'NONE',  ( -0.000000000000000000, -0.000000000000000000, 1.000000000000000000 ) ) ;
#9206=EDGE_CURVE ( 'NONE', #44135, #23261, #18163, .T. ) ;
#9208=CARTESIAN_POINT ( 'NONE',  ( 9.202092513630264312E-14, 200.0000000000001421, 0.000000000000000000 ) ) ;
#9329=VERTEX_POINT ( 'NONE', #22278 ) ;
#9331=VERTEX_POINT ( 'NONE', #18389 ) ;
#9357=CARTESIAN_POINT ( 'NONE',  ( 521.6730038022808458, 239.9999999999999432, -122.7905160835442615 ) ) ;
#9373=LINE ( 'NONE', #16071, #43188 ) ;
#9382=ORIENTED_EDGE ( 'NONE', *, *, #30289, .F. ) ;
#9428=VERTEX_POINT ( 'NONE', #28999 ) ;
#9445=EDGE_CURVE ( 'NONE', #43744, #44135, #14700, .T. ) ;
#9497=FACE_OUTER_BOUND ( 'NONE', #34391, .T. ) ;
#9541=CARTESIAN_POINT ( 'NONE',  ( -728.8365100919714905, 260.0000000000001705, -199.9999999999890861 ) ) ;
#9559=ORIENTED_EDGE ( 'NONE', *, *, #36894, .T. ) ;
#9567=DIRECTION ( 'NONE',  ( -0.000000000000000000, 1.000000000000000000, -0.000000000000000000 ) ) ;
#9623=CARTESIAN_POINT ( 'NONE',  ( 441.1634899080286232, 259.9999999999999432, -199.9999999999972431 ) ) ;
#9635=VERTEX_POINT ( 'NONE', #37274 ) ;
#9650=FACE_BOUND ( 'NONE', #11495, .T. ) ;
#9656=LINE ( 'NONE', #23719, #28482 ) ;
#9663=ORIENTED_EDGE ( 'NONE', *, *, #1807, .F. ) ;
#9678=DIRECTION ( 'NONE',  ( -0.000000000000000000, 1.000000000000000000, -0.000000000000000000 ) ) ;
#9694=DIRECTION ( 'NONE',  ( 1.000000000000000000, 0.000000000000000000, 0.000000000000000000 ) ) ;
#9744=AXIS2_PLACEMENT_3D ( 'NONE', #29466, #36167, #11233 ) ;
#9751=LINE ( 'NONE', #29692, #12450 ) ;
#9755=CARTESIAN_POINT ( 'NONE',  ( -468.8365100919714337, 260.0000000000001705, -202.7499999999907345 ) ) ;
#9868=AXIS2_PLACEMENT_3D ( 'NONE', #999, #4263, #1231 ) ;
#9882=AXIS2_PLACEMENT_3D ( 'NONE', #85, #28246, #42345 ) ;
#9894=AXIS2_PLACEMENT_3D ( 'NONE', #41455, #2882, #45382 ) ;
#9936=ORIENTED_EDGE ( 'NONE', *, *, #13763, .T. ) ;
#9939=PRODUCT_DEFINITION_CONTEXT ( 'detailed design', #22838, 'design' ) ;
#9950=VECTOR ( 'NONE', #33385, 1000.000000000000000 ) ;
#9985=LINE ( 'NONE', #45, #38003 ) ;
#10007=AXIS2_PLACEMENT_3D ( 'NONE', #9623, #23685, #37796 ) ;
#10075=VERTEX_POINT ( 'NONE', #38202 ) ;
#10092=FACE_OUTER_BOUND ( 'NONE', #7760, .T. ) ;
#10098=CARTESIAN_POINT ( 'NONE',  ( -78.83651009197140525, 240.0000000000000853, -197.2499999999937756 ) ) ;
#10142=CARTESIAN_POINT ( 'NONE',  ( 831.1634899080286232, 259.9999999999998863, -202.7499999999998295 ) ) ;
#10227=VERTEX_POINT ( 'NONE', #31494 ) ;
#10235=ORIENTED_EDGE ( 'NONE', *, *, #10256, .T. ) ;
#10256=EDGE_CURVE ( 'NONE', #22008, #7346, #10464, .T. ) ;
#10302=EDGE_CURVE ( 'NONE', #12556, #30518, #13030, .T. ) ;
#10315=DIRECTION ( 'NONE',  ( -1.880165489482579047E-16, -1.000000000000000000, -0.000000000000000000 ) ) ;
#10331=FACE_BOUND ( 'NONE', #30063, .T. ) ;
#10332=ADVANCED_FACE ( 'NONE', ( #31932 ), #11387, .F. ) ;
#10345=VERTEX_POINT ( 'NONE', #35184 ) ;
#10363=EDGE_CURVE ( 'NONE', #33702, #24407, #42802, .T. ) ;
#10441=LINE ( 'NONE', #34478, #15888 ) ;
#10464=LINE ( 'NONE', #24540, #4156 ) ;
#10474=CARTESIAN_POINT ( 'NONE',  ( -928.0249999999991815, 154.9999999999998863, 339.9999999999999432 ) ) ;
#10523=VERTEX_POINT ( 'NONE', #11626 ) ;
#10530=CARTESIAN_POINT ( 'NONE',  ( -338.8365100919713200, 260.0000000000001137, -199.9999999999917861 ) ) ;
#10547=EDGE_LOOP ( 'NONE', ( #22370, #23386, #17959, #41159 ) ) ;
#10556=EDGE_CURVE ( 'NONE', #791, #17477, #4861, .T. ) ;
#10582=DIRECTION ( 'NONE',  ( 0.000000000000000000, -1.000000000000000000, 0.000000000000000000 ) ) ;
#10612=FACE_BOUND ( 'NONE', #1586, .T. ) ;
#10692=CLOSED_SHELL ( 'NONE', ( #34665, #21512, #44723, #9179, #42193, #24287, #26631, #36769, #45562, #33708, #10332, #36262, #26653, #15081, #14248, #31158, #29498, #21901, #11437, #38, #37254, #38506, #29769, #767, #5814, #28002, #21517, #39693, #15643, #42762, #39136, #19695, #17082, #31933, #32949, #37413, #12026, #41653, #26383, #45627, #26718, #40817, #29218, #1589, #38741, #15626, #15679, #45490, #913, #44503, #40448, #35661, #28676, #42262 ) ) ;
#10717=VECTOR ( 'NONE', #22924, 1000.000000000000000 ) ;
#10735=VECTOR ( 'NONE', #27395, 1000.000000000000000 ) ;
#10758=ORIENTED_EDGE ( 'NONE', *, *, #31393, .F. ) ;
#10764=CARTESIAN_POINT ( 'NONE',  ( 949.5497976682736407, 229.9999999999998579, -2132.806278688367456 ) ) ;
#10786=VECTOR ( 'NONE', #33904, 1000.000000000000000 ) ;
#10809=AXIS2_PLACEMENT_3D ( 'NONE', #5397, #34037, #36833 ) ;
#10825=LINE ( 'NONE', #6887, #12792 ) ;
#10837=ORIENTED_EDGE ( 'NONE', *, *, #21886, .F. ) ;
#10887=LINE ( 'NONE', #36050, #3208 ) ;
#10888=EDGE_CURVE ( 'NONE', #28460, #5848, #40260, .T. ) ;
#10908=CARTESIAN_POINT ( 'NONE',  ( -338.8365100919713200, 230.0000000000001137, -199.9999999999917861 ) ) ;
#10945=LINE ( 'NONE', #21780, #7898 ) ;
#10953=VECTOR ( 'NONE', #42422, 1000.000000000000000 ) ;
#10969=DIRECTION ( 'NONE',  ( -0.000000000000000000, 1.000000000000000000, -0.000000000000000000 ) ) ;
#10975=FACE_OUTER_BOUND ( 'NONE', #39449, .T. ) ;
#10983=CARTESIAN_POINT ( 'NONE',  ( -521.6730038022808458, 200.0000000000001421, 339.9999999999999432 ) ) ;
#11019=AXIS2_PLACEMENT_3D ( 'NONE', #20317, #43886, #2300 ) ;
#11054=CARTESIAN_POINT ( 'NONE',  ( 571.1634899080285095, 259.9999999999999432, -202.7499999999980105 ) ) ;
#11058=DIRECTION ( 'NONE',  ( 0.000000000000000000, -0.000000000000000000, 1.000000000000000000 ) ) ;
#11101=ORIENTED_EDGE ( 'NONE', *, *, #43788, .T. ) ;
#11158=VERTEX_POINT ( 'NONE', #34446 ) ;
#11168=ORIENTED_EDGE ( 'NONE', *, *, #10888, .F. ) ;
#11203=DIRECTION ( 'NONE',  ( -1.880165489482579047E-16, -1.000000000000000000, -0.000000000000000000 ) ) ;
#11228=LINE ( 'NONE', #1282, #39660 ) ;
#11233=DIRECTION ( 'NONE',  ( 1.000000000000000000, 0.000000000000000000, 0.000000000000000000 ) ) ;
#11359=CIRCLE ( 'NONE', #23860, 2.749999999999863665 ) ;
#11387=CYLINDRICAL_SURFACE ( 'NONE', #1168, 2.749999999999863665 ) ;
#11389=VECTOR ( 'NONE', #12073, 1000.000000000000000 ) ;
#11398=DIRECTION ( 'NONE',  ( -1.880165489482579047E-16, -1.000000000000000000, -0.000000000000000000 ) ) ;
#11404=CARTESIAN_POINT ( 'NONE',  ( 521.6730038022808458, 230.0000000000002274, 339.9999999999999432 ) ) ;
#11414=DIRECTION ( 'NONE',  ( -1.000000000000000000, 0.000000000000000000, -0.000000000000000000 ) ) ;
#11437=ADVANCED_FACE ( 'NONE', ( #11518 ), #18230, .F. ) ;
#11447=CARTESIAN_POINT ( 'NONE',  ( 949.5497976682736407, 239.9999999999998863, 339.9999999999998863 ) ) ;
#11456=FACE_OUTER_BOUND ( 'NONE', #16847, .T. ) ;
#11495=EDGE_LOOP ( 'NONE', ( #26853, #37093 ) ) ;
#11518=FACE_OUTER_BOUND ( 'NONE', #30107, .T. ) ;
#11526=VERTEX_POINT ( 'NONE', #42693 ) ;
#11549=CIRCLE ( 'NONE', #24782, 2.749999999999863665 ) ;
#11563=ORIENTED_EDGE ( 'NONE', *, *, #12547, .F. ) ;
#11602=CIRCLE ( 'NONE', #17504, 2.749999999999835687 ) ;
#11614=EDGE_LOOP ( 'NONE', ( #37688, #10758 ) ) ;
#11622=ORIENTED_EDGE ( 'NONE', *, *, #10556, .F. ) ;
#11626=CARTESIAN_POINT ( 'NONE',  ( 831.1634899080286232, 229.9999999999998863, -202.7499999999998295 ) ) ;
#11630=EDGE_LOOP ( 'NONE', ( #305, #9936 ) ) ;
#11642=LINE ( 'NONE', #8175, #8427 ) ;
#11659=ORIENTED_EDGE ( 'NONE', *, *, #44442, .F. ) ;
#11713=DIRECTION ( 'NONE',  ( 1.000000000000000000, 0.000000000000000000, 0.000000000000000000 ) ) ;
#11769=ORIENTED_EDGE ( 'NONE', *, *, #18712, .T. ) ;
#11775=AXIS2_PLACEMENT_3D ( 'NONE', #15213, #23167, #33817 ) ;
#11848=ORIENTED_EDGE ( 'NONE', *, *, #4927, .F. ) ;
#11884=DIRECTION ( 'NONE',  ( -1.880165489482579047E-16, -1.000000000000000000, -0.000000000000000000 ) ) ;
#11886=ORIENTED_EDGE ( 'NONE', *, *, #2160, .F. ) ;
#11899=CIRCLE ( 'NONE', #31801, 2.749999999999863665 ) ;
#11911=LINE ( 'NONE', #19509, #17996 ) ;
#11925=ORIENTED_EDGE ( 'NONE', *, *, #41944, .F. ) ;
#11961=CARTESIAN_POINT ( 'NONE',  ( -959.5497976682736407, 240.0000000000002274, -209.9999999999999716 ) ) ;
#11975=ORIENTED_EDGE ( 'NONE', *, *, #5499, .F. ) ;
#11989=DIRECTION ( 'NONE',  ( -1.880165489482579047E-16, -1.000000000000000000, -0.000000000000000000 ) ) ;
#12012=ORIENTED_EDGE ( 'NONE', *, *, #22981, .T. ) ;
#12026=ADVANCED_FACE ( 'NONE', ( #38043 ), #31564, .F. ) ;
#12068=MECHANICAL_DESIGN_GEOMETRIC_PRESENTATION_REPRESENTATION('',(#20883),#41569);
#12073=DIRECTION ( 'NONE',  ( 1.880165489482579047E-16, 1.000000000000000000, 0.000000000000000000 ) ) ;
#12086=AXIS2_PLACEMENT_3D ( 'NONE', #15102, #7715, #29192 ) ;
#12093=PLANE ( 'NONE',  #22449 ) ;
#12108=VERTEX_POINT ( 'NONE', #41967 ) ;
#12135=CARTESIAN_POINT ( 'NONE',  ( -919.9999999999993179, 219.9999999999998863, 350.0000000000000000 ) ) ;
#12147=CARTESIAN_POINT ( 'NONE',  ( -338.8365100919713200, 230.0000000000001137, -199.9999999999917861 ) ) ;
#12154=DIRECTION ( 'NONE',  ( 1.000000000000000000, 0.000000000000000000, 0.000000000000000000 ) ) ;
#12158=ORIENTED_EDGE ( 'NONE', *, *, #37965, .T. ) ;
#12192=DIRECTION ( 'NONE',  ( -1.000000000000000000, 0.000000000000000000, 0.000000000000000000 ) ) ;
#12214=VECTOR ( 'NONE', #2393, 1000.000000000000000 ) ;
#12248=ORIENTED_EDGE ( 'NONE', *, *, #18500, .F. ) ;
#12262=EDGE_CURVE ( 'NONE', #19031, #19590, #42451, .T. ) ;
#12304=DIRECTION ( 'NONE',  ( 1.000000000000000000, 0.000000000000000000, 0.000000000000000000 ) ) ;
#12316=LINE ( 'NONE', #22912, #5506 ) ;
#12326=PLANE ( 'NONE',  #32808 ) ;
#12336=VECTOR ( 'NONE', #21613, 1000.000000000000000 ) ;
#12362=AXIS2_PLACEMENT_3D ( 'NONE', #15127, #4501, #28984 ) ;
#12366=CARTESIAN_POINT ( 'NONE',  ( 521.6730038022808458, -9.808315785437627339E-14, 350.0000000000000000 ) ) ;
#12388=EDGE_LOOP ( 'NONE', ( #6316, #12613, #26870, #29525 ) ) ;
#12406=DIRECTION ( 'NONE',  ( 1.880165489482579047E-16, 1.000000000000000000, -0.000000000000000000 ) ) ;
#12417=LINE ( 'NONE', #5249, #31882 ) ;
#12450=VECTOR ( 'NONE', #43768, 1000.000000000000000 ) ;
#12500=ORIENTED_EDGE ( 'NONE', *, *, #10302, .F. ) ;
#12513=VECTOR ( 'NONE', #38424, 1000.000000000000000 ) ;
#12526=CARTESIAN_POINT ( 'NONE',  ( -858.8365100919713768, 260.0000000000002274, -199.9999999999881481 ) ) ;
#12539=CARTESIAN_POINT ( 'NONE',  ( -959.5497976682736407, 240.0000000000002274, -209.9999999999999716 ) ) ;
#12547=EDGE_CURVE ( 'NONE', #42970, #27381, #22286, .T. ) ;
#12556=VERTEX_POINT ( 'NONE', #43092 ) ;
#12613=ORIENTED_EDGE ( 'NONE', *, *, #21855, .T. ) ;
#12642=CARTESIAN_POINT ( 'NONE',  ( 949.5497976682736407, 229.9999999999998579, 339.9999999999999432 ) ) ;
#12654=ORIENTED_EDGE ( 'NONE', *, *, #15853, .T. ) ;
#12657=CARTESIAN_POINT ( 'NONE',  ( -928.0249999999991815, 219.9999999999998863, 350.0000000000000000 ) ) ;
#12697=VECTOR ( 'NONE', #9678, 1000.000000000000000 ) ;
#12718=VERTEX_POINT ( 'NONE', #32697 ) ;
#12737=CARTESIAN_POINT ( 'NONE',  ( -728.8365100919714905, 230.0000000000001705, -202.7499999999889440 ) ) ;
#12742=DIRECTION ( 'NONE',  ( 1.000000000000000000, 0.000000000000000000, 0.000000000000000000 ) ) ;
#12788=VERTEX_POINT ( 'NONE', #35464 ) ;
#12792=VECTOR ( 'NONE', #13836, 1000.000000000000000 ) ;
#12824=FACE_OUTER_BOUND ( 'NONE', #21247, .T. ) ;
#12852=CARTESIAN_POINT ( 'NONE',  ( 181.1634899080285948, 260.0000000000000000, -197.2499999999955662 ) ) ;
#12861=DIRECTION ( 'NONE',  ( 1.000000000000000000, 0.000000000000000000, 0.000000000000000000 ) ) ;
#12866=DIRECTION ( 'NONE',  ( -0.000000000000000000, 1.000000000000000000, -0.000000000000000000 ) ) ;
#12970=ORIENTED_EDGE ( 'NONE', *, *, #6919, .T. ) ;
#13030=LINE ( 'NONE', #41211, #24772 ) ;
#13047=CIRCLE ( 'NONE', #35926, 8.024999999999948841 ) ;
#13091=CIRCLE ( 'NONE', #3495, 2.749999999999835687 ) ;
#13111=ORIENTED_EDGE ( 'NONE', *, *, #33150, .F. ) ;
#13142=VERTEX_POINT ( 'NONE', #37046 ) ;
#13155=EDGE_CURVE ( 'NONE', #9635, #39962, #21126, .T. ) ;
#13230=DIRECTION ( 'NONE',  ( 1.000000000000000000, 0.000000000000000000, 0.000000000000000000 ) ) ;
#13253=VERTEX_POINT ( 'NONE', #30344 ) ;
#13258=ORIENTED_EDGE ( 'NONE', *, *, #30571, .T. ) ;
#13283=DIRECTION ( 'NONE',  ( -1.880165489482579047E-16, -1.000000000000000000, 0.000000000000000000 ) ) ;
#13303=CARTESIAN_POINT ( 'NONE',  ( 181.1634899080285948, 230.0000000000000000, -199.9999999999953957 ) ) ;
#13326=DIRECTION ( 'NONE',  ( 0.000000000000000000, 0.000000000000000000, 1.000000000000000000 ) ) ;
#13330=DIRECTION ( 'NONE',  ( -1.000000000000000000, 0.000000000000000000, -0.000000000000000000 ) ) ;
#13336=DIRECTION ( 'NONE',  ( -1.880165489482579047E-16, -1.000000000000000000, -0.000000000000000000 ) ) ;
#13357=ORIENTED_EDGE ( 'NONE', *, *, #26058, .T. ) ;
#13384=ORIENTED_EDGE ( 'NONE', *, *, #5499, .T. ) ;
#13433=EDGE_CURVE ( 'NONE', #34173, #45635, #38207, .T. ) ;
#13475=ORIENTED_EDGE ( 'NONE', *, *, #29751, .F. ) ;
#13538=VERTEX_POINT ( 'NONE', #13950 ) ;
#13566=CYLINDRICAL_SURFACE ( 'NONE', #24942, 2.749999999999863665 ) ;
#13620=LINE ( 'NONE', #38338, #15871 ) ;
#13659=AXIS2_PLACEMENT_3D ( 'NONE', #42767, #42992, #18309 ) ;
#13702=AXIS2_PLACEMENT_3D ( 'NONE', #42588, #31498, #21549 ) ;
#13713=ORIENTED_EDGE ( 'NONE', *, *, #35022, .T. ) ;
#13716=ORIENTED_EDGE ( 'NONE', *, *, #15084, .F. ) ;
#13732=DIRECTION ( 'NONE',  ( 0.000000000000000000, 0.000000000000000000, 1.000000000000000000 ) ) ;
#13751=CARTESIAN_POINT ( 'NONE',  ( 181.1634899080285948, 260.0000000000000000, -202.7499999999952536 ) ) ;
#13757=EDGE_CURVE ( 'NONE', #3427, #32578, #41439, .T. ) ;
#13761=ORIENTED_EDGE ( 'NONE', *, *, #22981, .F. ) ;
#13763=EDGE_CURVE ( 'NONE', #24071, #44488, #7888, .T. ) ;
#13769=VERTEX_POINT ( 'NONE', #19388 ) ;
#13786=ORIENTED_EDGE ( 'NONE', *, *, #39132, .T. ) ;
#13798=CARTESIAN_POINT ( 'NONE',  ( 441.1634899080286232, 240.0000000000000000, -202.7499999999971010 ) ) ;
#13809=ORIENTED_EDGE ( 'NONE', *, *, #1475, .F. ) ;
#13816=ORIENTED_EDGE ( 'NONE', *, *, #14766, .T. ) ;
#13836=DIRECTION ( 'NONE',  ( -0.000000000000000000, 1.000000000000000000, -0.000000000000000000 ) ) ;
#13872=ORIENTED_EDGE ( 'NONE', *, *, #12547, .T. ) ;
#13878=ORIENTED_EDGE ( 'NONE', *, *, #16833, .T. ) ;
#13941=CIRCLE ( 'NONE', #41979, 2.749999999999863665 ) ;
#13950=CARTESIAN_POINT ( 'NONE',  ( -959.5497976682736407, 120.6654763175833693, -209.9999999999999716 ) ) ;
#13984=ORIENTED_EDGE ( 'NONE', *, *, #44480, .F. ) ;
#14006=CYLINDRICAL_SURFACE ( 'NONE', #10007, 2.749999999999863665 ) ;
#14070=DIRECTION ( 'NONE',  ( 1.000000000000000000, 0.000000000000000000, 0.000000000000000000 ) ) ;
#14149=ORIENTED_EDGE ( 'NONE', *, *, #41924, .F. ) ;
#14178=DIRECTION ( 'NONE',  ( -1.880165489482579047E-16, -1.000000000000000000, -0.000000000000000000 ) ) ;
#14201=DIRECTION ( 'NONE',  ( -0.000000000000000000, -0.000000000000000000, -1.000000000000000000 ) ) ;
#14235=CARTESIAN_POINT ( 'NONE',  ( 571.1634899080285095, 239.9999999999999716, -199.9999999999981526 ) ) ;
#14248=ADVANCED_FACE ( 'NONE', ( #27452 ), #20531, .F. ) ;
#14293=CARTESIAN_POINT ( 'NONE',  ( 441.1634899080286232, 240.0000000000000000, -199.9999999999972431 ) ) ;
#14313=FACE_BOUND ( 'NONE', #37627, .T. ) ;
#14331=VERTEX_POINT ( 'NONE', #3678 ) ;
#14389=EDGE_LOOP ( 'NONE', ( #25327, #28409, #718, #804, #33351, #7200 ) ) ;
#14391=EDGE_LOOP ( 'NONE', ( #21314, #3770 ) ) ;
#14416=LINE ( 'NONE', #28732, #36423 ) ;
#14495=CARTESIAN_POINT ( 'NONE',  ( 571.1634899080285095, 229.9999999999999432, -202.7499999999980105 ) ) ;
#14595=ORIENTED_EDGE ( 'NONE', *, *, #44639, .F. ) ;
#14605=EDGE_CURVE ( 'NONE', #10227, #5810, #1107, .T. ) ;
#14615=EDGE_CURVE ( 'NONE', #24672, #40820, #14982, .T. ) ;
#14652=EDGE_LOOP ( 'NONE', ( #23449, #20893 ) ) ;
#14669=CARTESIAN_POINT ( 'NONE',  ( -728.8365100919714905, 240.0000000000001990, -197.2499999999891998 ) ) ;
#14678=ORIENTED_EDGE ( 'NONE', *, *, #40553, .F. ) ;
#14684=ORIENTED_EDGE ( 'NONE', *, *, #39673, .T. ) ;
#14700=LINE ( 'NONE', #10764, #25504 ) ;
#14734=VERTEX_POINT ( 'NONE', #35761 ) ;
#14766=EDGE_CURVE ( 'NONE', #12788, #15138, #13047, .T. ) ;
#14797=ORIENTED_EDGE ( 'NONE', *, *, #12262, .T. ) ;
#14822=DIRECTION ( 'NONE',  ( -0.000000000000000000, 1.000000000000000000, -0.000000000000000000 ) ) ;
#14838=PLANE ( 'NONE',  #13659 ) ;
#14856=VERTEX_POINT ( 'NONE', #11961 ) ;
#14870=DIRECTION ( 'NONE',  ( -0.000000000000000000, -0.000000000000000000, -1.000000000000000000 ) ) ;
#14896=CARTESIAN_POINT ( 'NONE',  ( -858.8365100919713768, 230.0000000000001990, -199.9999999999881481 ) ) ;
#14930=FACE_OUTER_BOUND ( 'NONE', #14389, .T. ) ;
#14949=ORIENTED_EDGE ( 'NONE', *, *, #13155, .T. ) ;
#14982=LINE ( 'NONE', #18233, #27086 ) ;
#14993=CIRCLE ( 'NONE', #21610, 2.749999999999842792 ) ;
#15000=ORIENTED_EDGE ( 'NONE', *, *, #39742, .F. ) ;
#15004=LINE ( 'NONE', #8531, #10786 ) ;
#15014=VERTEX_POINT ( 'NONE', #27188 ) ;
#15020=AXIS2_PLACEMENT_3D ( 'NONE', #27913, #24430, #21438 ) ;
#15039=CIRCLE ( 'NONE', #37171, 2.749999999999835687 ) ;
#15048=CARTESIAN_POINT ( 'NONE',  ( 454.7528517110262101, 199.9999999999999432, -122.7905160835442615 ) ) ;
#15069=DIRECTION ( 'NONE',  ( -0.000000000000000000, -0.000000000000000000, 1.000000000000000000 ) ) ;
#15073=ORIENTED_EDGE ( 'NONE', *, *, #35323, .T. ) ;
#15081=ADVANCED_FACE ( 'NONE', ( #20245 ), #26497, .F. ) ;
#15084=EDGE_CURVE ( 'NONE', #35455, #15202, #5710, .T. ) ;
#15087=DIRECTION ( 'NONE',  ( 1.000000000000000000, 0.000000000000000000, 0.000000000000000000 ) ) ;
#15102=CARTESIAN_POINT ( 'NONE',  ( 571.1634899080285095, 259.9999999999999432, -199.9999999999981526 ) ) ;
#15110=DIRECTION ( 'NONE',  ( 0.000000000000000000, 0.000000000000000000, 1.000000000000000000 ) ) ;
#15118=CARTESIAN_POINT ( 'NONE',  ( 919.9999999999993179, 154.9999999999998863, -360.0000000000000000 ) ) ;
#15127=CARTESIAN_POINT ( 'NONE',  ( -919.9999999999993179, 219.9999999999998863, 339.9999999999999432 ) ) ;
#15133=ORIENTED_EDGE ( 'NONE', *, *, #17129, .T. ) ;
#15138=VERTEX_POINT ( 'NONE', #30879 ) ;
#15145=DIRECTION ( 'NONE',  ( 1.000000000000000000, 0.000000000000000000, 0.000000000000000000 ) ) ;
#15174=FACE_OUTER_BOUND ( 'NONE', #26172, .T. ) ;
#15190=( LENGTH_UNIT ( ) NAMED_UNIT ( * ) SI_UNIT ( .MILLI., .METRE. ) );
#15202=VERTEX_POINT ( 'NONE', #34096 ) ;
#15213=CARTESIAN_POINT ( 'NONE',  ( 701.1634899080286232, 259.9999999999999432, -199.9999999999990337 ) ) ;
#15229=CARTESIAN_POINT ( 'NONE',  ( -949.5497976682736407, 230.0000000000002274, -210.0000000000000000 ) ) ;
#15253=ORIENTED_EDGE ( 'NONE', *, *, #25811, .F. ) ;
#15260=VERTEX_POINT ( 'NONE', #19797 ) ;
#15268=VECTOR ( 'NONE', #20181, 1000.000000000000000 ) ;
#15281=DIRECTION ( 'NONE',  ( 0.000000000000000000, 0.000000000000000000, 1.000000000000000000 ) ) ;
#15331=LINE ( 'NONE', #32430, #18634 ) ;
#15382=CARTESIAN_POINT ( 'NONE',  ( -454.7528517110260964, 230.0000000000001421, -122.7905160835438068 ) ) ;
#15387=LINE ( 'NONE', #35941, #25958 ) ;
#15404=AXIS2_PLACEMENT_3D ( 'NONE', #35263, #29264, #35955 ) ;
#15406=DIRECTION ( 'NONE',  ( -1.880165489482579047E-16, -1.000000000000000000, -0.000000000000000000 ) ) ;
#15485=EDGE_LOOP ( 'NONE', ( #28941, #2632, #14678, #29895 ) ) ;
#15534=VERTEX_POINT ( 'NONE', #13798 ) ;
#15541=CARTESIAN_POINT ( 'NONE',  ( -468.8365100919714337, 240.0000000000001705, -202.7499999999907345 ) ) ;
#15542=ORIENTED_EDGE ( 'NONE', *, *, #39901, .T. ) ;
#15549=DIRECTION ( 'NONE',  ( 1.000000000000000000, 0.000000000000000000, 0.000000000000000000 ) ) ;
#15558=FACE_OUTER_BOUND ( 'NONE', #27000, .T. ) ;
#15575=EDGE_CURVE ( 'NONE', #9331, #6874, #39681, .T. ) ;
#15617=ORIENTED_EDGE ( 'NONE', *, *, #5541, .T. ) ;
#15626=ADVANCED_FACE ( 'NONE', ( #38045 ), #41739, .F. ) ;
#15643=ADVANCED_FACE ( 'NONE', ( #10092 ), #45435, .F. ) ;
#15673=CIRCLE ( 'NONE', #41495, 2.749999999999863665 ) ;
#15679=ADVANCED_FACE ( 'NONE', ( #14930 ), #4528, .F. ) ;
#15735=AXIS2_PLACEMENT_3D ( 'NONE', #19133, #40823, #5717 ) ;
#15737=ORIENTED_EDGE ( 'NONE', *, *, #40568, .T. ) ;
#15763=FACE_OUTER_BOUND ( 'NONE', #3304, .T. ) ;
#15766=AXIS2_PLACEMENT_3D ( 'NONE', #45200, #13336, #17248 ) ;
#15775=FACE_BOUND ( 'NONE', #36415, .T. ) ;
#15805=ORIENTED_EDGE ( 'NONE', *, *, #26636, .T. ) ;
#15837=DIRECTION ( 'NONE',  ( 1.000000000000000000, 0.000000000000000000, 0.000000000000000000 ) ) ;
#15853=EDGE_CURVE ( 'NONE', #33957, #15534, #15387, .T. ) ;
#15871=VECTOR ( 'NONE', #6220, 1000.000000000000000 ) ;
#15875=DIRECTION ( 'NONE',  ( 0.000000000000000000, 1.000000000000000000, 0.000000000000000000 ) ) ;
#15877=EDGE_CURVE ( 'NONE', #23028, #40984, #9015, .T. ) ;
#15888=VECTOR ( 'NONE', #23604, 1000.000000000000000 ) ;
#15903=VECTOR ( 'NONE', #28295, 1000.000000000000000 ) ;
#15928=DIRECTION ( 'NONE',  ( -0.000000000000000000, -0.000000000000000000, 1.000000000000000000 ) ) ;
#15974=ORIENTED_EDGE ( 'NONE', *, *, #23535, .F. ) ;
#15979=ORIENTED_EDGE ( 'NONE', *, *, #10888, .T. ) ;
#15988=AXIS2_PLACEMENT_3D ( 'NONE', #925, #38843, #3945 ) ;
#15992=DIRECTION ( 'NONE',  ( -1.000000000000000000, 0.000000000000000000, 0.000000000000000000 ) ) ;
#16011=FACE_BOUND ( 'NONE', #11614, .T. ) ;
#16038=CARTESIAN_POINT ( 'NONE',  ( -78.83651009197140525, 240.0000000000000853, -202.7499999999934346 ) ) ;
#16071=CARTESIAN_POINT ( 'NONE',  ( 521.6730038022808458, 199.9999999999999147, -122.7905160835442615 ) ) ;
#16121=DIRECTION ( 'NONE',  ( 0.000000000000000000, 0.000000000000000000, 1.000000000000000000 ) ) ;
#16146=ORIENTED_EDGE ( 'NONE', *, *, #9445, .T. ) ;
#16168=LINE ( 'NONE', #30250, #23962 ) ;
#16171=AXIS2_PLACEMENT_3D ( 'NONE', #18445, #29301, #22119 ) ;
#16185=EDGE_CURVE ( 'NONE', #5955, #20856, #8684, .T. ) ;
#16189=ORIENTED_EDGE ( 'NONE', *, *, #15084, .T. ) ;
#16208=DIRECTION ( 'NONE',  ( 0.000000000000000000, 0.000000000000000000, 1.000000000000000000 ) ) ;
#16245=ORIENTED_EDGE ( 'NONE', *, *, #4645, .T. ) ;
#16293=LINE ( 'NONE', #30375, #32074 ) ;
#16308=EDGE_CURVE ( 'NONE', #30518, #11526, #3119, .T. ) ;
#16428=AXIS2_PLACEMENT_3D ( 'NONE', #17938, #3630, #39194 ) ;
#16434=DIRECTION ( 'NONE',  ( 1.000000000000000000, -4.147566128926370535E-16, 0.000000000000000000 ) ) ;
#16441=DIRECTION ( 'NONE',  ( -1.880165489482579047E-16, -1.000000000000000000, -0.000000000000000000 ) ) ;
#16570=EDGE_CURVE ( 'NONE', #38643, #11526, #88, .T. ) ;
#16598=ORIENTED_EDGE ( 'NONE', *, *, #42492, .T. ) ;
#16603=VERTEX_POINT ( 'NONE', #42126 ) ;
#16658=PLANE ( 'NONE',  #22729 ) ;
#16702=CARTESIAN_POINT ( 'NONE',  ( 959.5497976682736407, 239.9999999999998863, -209.9999999999999716 ) ) ;
#16715=DIRECTION ( 'NONE',  ( -1.000000000000000000, 4.147566128926370535E-16, -0.000000000000000000 ) ) ;
#16749=PLANE ( 'NONE',  #38659 ) ;
#16791=EDGE_CURVE ( 'NONE', #13142, #15014, #1658, .T. ) ;
#16815=ORIENTED_EDGE ( 'NONE', *, *, #33150, .T. ) ;
#16833=EDGE_CURVE ( 'NONE', #14734, #5955, #15331, .T. ) ;
#16847=EDGE_LOOP ( 'NONE', ( #23409, #9083, #4343, #5870 ) ) ;
#16881=EDGE_LOOP ( 'NONE', ( #5694, #20625 ) ) ;
#16898=ORIENTED_EDGE ( 'NONE', *, *, #13433, .T. ) ;
#16902=CARTESIAN_POINT ( 'NONE',  ( 8.295132257852746908E-14, 200.0000000000001421, 339.9999999999999432 ) ) ;
#16918=CARTESIAN_POINT ( 'NONE',  ( 311.1634899080286232, 240.0000000000000000, -199.9999999999963336 ) ) ;
#16933=VERTEX_POINT ( 'NONE', #18790 ) ;
#16940=ORIENTED_EDGE ( 'NONE', *, *, #8086, .F. ) ;
#16946=ORIENTED_EDGE ( 'NONE', *, *, #15877, .F. ) ;
#16953=DIRECTION ( 'NONE',  ( -1.880165489482579047E-16, -1.000000000000000000, -0.000000000000000000 ) ) ;
#16958=EDGE_LOOP ( 'NONE', ( #38904, #16245 ) ) ;
#16973=CARTESIAN_POINT ( 'NONE',  ( -338.8365100919713200, 240.0000000000001421, -199.9999999999917861 ) ) ;
#17049=EDGE_CURVE ( 'NONE', #24181, #16933, #11899, .T. ) ;
#17082=ADVANCED_FACE ( 'NONE', ( #15763 ), #1891, .F. ) ;
#17085=DIRECTION ( 'NONE',  ( -1.880165489482579047E-16, -1.000000000000000000, -0.000000000000000000 ) ) ;
#17111=EDGE_CURVE ( 'NONE', #15260, #40820, #824, .T. ) ;
#17129=EDGE_CURVE ( 'NONE', #39820, #1382, #6715, .T. ) ;
#17177=ORIENTED_EDGE ( 'NONE', *, *, #8086, .T. ) ;
#17248=DIRECTION ( 'NONE',  ( 1.000000000000000000, 0.000000000000000000, 0.000000000000000000 ) ) ;
#17262=VERTEX_POINT ( 'NONE', #5354 ) ;
#17267=ORIENTED_EDGE ( 'NONE', *, *, #39387, .T. ) ;
#17289=DIRECTION ( 'NONE',  ( 1.000000000000000000, -1.880165489482579047E-16, 0.000000000000000000 ) ) ;
#17308=DIRECTION ( 'NONE',  ( -0.000000000000000000, -0.000000000000000000, 1.000000000000000000 ) ) ;
#17344=ORIENTED_EDGE ( 'NONE', *, *, #32332, .T. ) ;
#17356=CARTESIAN_POINT ( 'NONE',  ( 51.16348990802859475, 260.0000000000000568, -197.2499999999946851 ) ) ;
#17428=CARTESIAN_POINT ( 'NONE',  ( -338.8365100919713200, 260.0000000000001137, -202.7499999999916724 ) ) ;
#17477=VERTEX_POINT ( 'NONE', #38605 ) ;
#17495=LINE ( 'NONE', #41978, #41588 ) ;
#17499=DIRECTION ( 'NONE',  ( -0.000000000000000000, 1.000000000000000000, -0.000000000000000000 ) ) ;
#17504=AXIS2_PLACEMENT_3D ( 'NONE', #17548, #39027, #21920 ) ;
#17544=ORIENTED_EDGE ( 'NONE', *, *, #5098, .F. ) ;
#17548=CARTESIAN_POINT ( 'NONE',  ( 181.1634899080285948, 240.0000000000000284, -199.9999999999953957 ) ) ;
#17584=CYLINDRICAL_SURFACE ( 'NONE', #24043, 2.749999999999835687 ) ;
#17668=EDGE_CURVE ( 'NONE', #9428, #32578, #43638, .T. ) ;
#17680=DIRECTION ( 'NONE',  ( -1.880165489482579047E-16, -1.000000000000000000, -0.000000000000000000 ) ) ;
#17690=ORIENTED_EDGE ( 'NONE', *, *, #15853, .F. ) ;
#17747=ORIENTED_EDGE ( 'NONE', *, *, #21824, .T. ) ;
#17769=EDGE_LOOP ( 'NONE', ( #17544, #13816, #15805, #36695 ) ) ;
#17867=ORIENTED_EDGE ( 'NONE', *, *, #31416, .F. ) ;
#17873=AXIS2_PLACEMENT_3D ( 'NONE', #45195, #31096, #27875 ) ;
#17881=CARTESIAN_POINT ( 'NONE',  ( 521.6730038022808458, 199.9999999999999147, -122.7905160835442615 ) ) ;
#17890=CARTESIAN_POINT ( 'NONE',  ( -208.8365100919714052, 240.0000000000001137, -202.7499999999925251 ) ) ;
#17892=VECTOR ( 'NONE', #39930, 1000.000000000000000 ) ;
#17897=DIRECTION ( 'NONE',  ( 1.000000000000000000, 0.000000000000000000, 0.000000000000000000 ) ) ;
#17905=DIRECTION ( 'NONE',  ( -1.000000000000000000, 0.000000000000000000, 0.000000000000000000 ) ) ;
#17914=ORIENTED_EDGE ( 'NONE', *, *, #27798, .T. ) ;
#17924=EDGE_CURVE ( 'NONE', #11158, #8116, #18795, .T. ) ;
#17932=CARTESIAN_POINT ( 'NONE',  ( 181.1634899080285948, 260.0000000000000000, -199.9999999999953957 ) ) ;
#17937=DIRECTION ( 'NONE',  ( 1.000000000000000000, 0.000000000000000000, 0.000000000000000000 ) ) ;
#17938=CARTESIAN_POINT ( 'NONE',  ( 919.9999999999993179, 219.9999999999998863, -360.0000000000000000 ) ) ;
#17957=EDGE_CURVE ( 'NONE', #15534, #44890, #34262, .T. ) ;
#17959=ORIENTED_EDGE ( 'NONE', *, *, #21824, .F. ) ;
#17966=ORIENTED_EDGE ( 'NONE', *, *, #3591, .T. ) ;
#17996=VECTOR ( 'NONE', #30363, 1000.000000000000000 ) ;
#18019=ORIENTED_EDGE ( 'NONE', *, *, #39979, .F. ) ;
#18120=FACE_OUTER_BOUND ( 'NONE', #39811, .T. ) ;
#18137=EDGE_LOOP ( 'NONE', ( #8977, #36899 ) ) ;
#18163=LINE ( 'NONE', #11447, #15903 ) ;
#18171=LINE ( 'NONE', #8216, #12336 ) ;
#18176=VECTOR ( 'NONE', #29190, 1000.000000000000000 ) ;
#18229=CARTESIAN_POINT ( 'NONE',  ( -454.7528517110260964, 200.0000000000001137, -122.7905160835438068 ) ) ;
#18230=PLANE ( 'NONE',  #3458 ) ;
#18233=CARTESIAN_POINT ( 'NONE',  ( 701.1634899080286232, 259.9999999999999432, -202.7499999999988916 ) ) ;
#18242=VECTOR ( 'NONE', #3452, 1000.000000000000000 ) ;
#18254=DIRECTION ( 'NONE',  ( 0.000000000000000000, 0.000000000000000000, 1.000000000000000000 ) ) ;
#18284=CARTESIAN_POINT ( 'NONE',  ( 701.1634899080286232, 229.9999999999999147, -202.7499999999988916 ) ) ;
#18296=CARTESIAN_POINT ( 'NONE',  ( -919.9999999999993179, 219.9999999999998863, 350.0000000000000000 ) ) ;
#18309=DIRECTION ( 'NONE',  ( -1.000000000000000000, 0.000000000000000000, -0.000000000000000000 ) ) ;
#18362=ORIENTED_EDGE ( 'NONE', *, *, #8497, .T. ) ;
#18389=CARTESIAN_POINT ( 'NONE',  ( 181.1634899080285948, 240.0000000000000284, -202.7499999999952536 ) ) ;
#18396=FACE_OUTER_BOUND ( 'NONE', #36935, .T. ) ;
#18418=CARTESIAN_POINT ( 'NONE',  ( 51.16348990802859475, 230.0000000000000284, -202.7499999999943441 ) ) ;
#18445=CARTESIAN_POINT ( 'NONE',  ( 959.5497976682736407, 239.9999999999998863, -2132.806278688367456 ) ) ;
#18448=ORIENTED_EDGE ( 'NONE', *, *, #44480, .T. ) ;
#18451=DIRECTION ( 'NONE',  ( 0.000000000000000000, 1.000000000000000000, 0.000000000000000000 ) ) ;
#18453=CARTESIAN_POINT ( 'NONE',  ( -521.6730038022809595, 230.0000000000001421, -2132.806278688367456 ) ) ;
#18500=EDGE_CURVE ( 'NONE', #5810, #26734, #42648, .T. ) ;
#18525=LINE ( 'NONE', #32606, #29161 ) ;
#18541=AXIS2_PLACEMENT_3D ( 'NONE', #26822, #16441, #8840 ) ;
#18543=ORIENTED_EDGE ( 'NONE', *, *, #22489, .F. ) ;
#18548=ORIENTED_EDGE ( 'NONE', *, *, #10556, .T. ) ;
#18561=CARTESIAN_POINT ( 'NONE',  ( -598.8365100919716042, 230.0000000000001421, -199.9999999999899671 ) ) ;
#18580=FACE_BOUND ( 'NONE', #24575, .T. ) ;
#18585=DIRECTION ( 'NONE',  ( 1.000000000000000000, 0.000000000000000000, 0.000000000000000000 ) ) ;
#18603=ORIENTED_EDGE ( 'NONE', *, *, #42189, .T. ) ;
#18620=DIRECTION ( 'NONE',  ( 1.000000000000000000, -1.880165489482579047E-16, 0.000000000000000000 ) ) ;
#18634=VECTOR ( 'NONE', #555, 1000.000000000000000 ) ;
#18645=ORIENTED_EDGE ( 'NONE', *, *, #13155, .F. ) ;
#18678=CARTESIAN_POINT ( 'NONE',  ( 949.5497976682736407, 239.9999999999998863, -2132.806278688367456 ) ) ;
#18712=EDGE_CURVE ( 'NONE', #36831, #14331, #8008, .T. ) ;
#18718=DIRECTION ( 'NONE',  ( -0.000000000000000000, -0.000000000000000000, 1.000000000000000000 ) ) ;
#18761=ORIENTED_EDGE ( 'NONE', *, *, #14605, .F. ) ;
#18779=DIRECTION ( 'NONE',  ( -0.000000000000000000, 0.000000000000000000, -1.000000000000000000 ) ) ;
#18790=CARTESIAN_POINT ( 'NONE',  ( 311.1634899080286232, 229.9999999999999716, -197.2499999999964473 ) ) ;
#18795=CIRCLE ( 'NONE', #21745, 2.749999999999835687 ) ;
#18815=ORIENTED_EDGE ( 'NONE', *, *, #37974, .T. ) ;
#18840=AXIS2_PLACEMENT_3D ( 'NONE', #44179, #5371, #5160 ) ;
#18869=AXIS2_PLACEMENT_3D ( 'NONE', #14896, #22252, #42368 ) ;
#18884=CIRCLE ( 'NONE', #24766, 2.749999999999919176 ) ;
#18887=VECTOR ( 'NONE', #25471, 1000.000000000000000 ) ;
#18903=SHAPE_REPRESENTATION ( 'Fixed Blade Support Base', ( #26858 ), #32022 ) ;
#18904=LINE ( 'NONE', #18229, #4911 ) ;
#18907=DIRECTION ( 'NONE',  ( 0.000000000000000000, 0.000000000000000000, -1.000000000000000000 ) ) ;
#18949=ORIENTED_EDGE ( 'NONE', *, *, #23149, .T. ) ;
#18954=CARTESIAN_POINT ( 'NONE',  ( 959.5497976682736407, 229.9999999999998579, 339.9999999999998863 ) ) ;
#18995=CIRCLE ( 'NONE', #28589, 8.024999999999948841 ) ;
#19031=VERTEX_POINT ( 'NONE', #20584 ) ;
#19133=CARTESIAN_POINT ( 'NONE',  ( 701.1634899080286232, 239.9999999999999432, -199.9999999999990337 ) ) ;
#19169=ORIENTED_EDGE ( 'NONE', *, *, #10363, .T. ) ;
#19189=LINE ( 'NONE', #15048, #43444 ) ;
#19240=DIRECTION ( 'NONE',  ( -0.000000000000000000, 0.000000000000000000, 1.000000000000000000 ) ) ;
#19256=CARTESIAN_POINT ( 'NONE',  ( 51.16348990802859475, 260.0000000000000568, -199.9999999999945146 ) ) ;
#19262=ORIENTED_EDGE ( 'NONE', *, *, #426, .F. ) ;
#19291=EDGE_CURVE ( 'NONE', #39949, #33570, #34897, .T. ) ;
#19339=DIRECTION ( 'NONE',  ( -0.000000000000000000, -0.000000000000000000, 1.000000000000000000 ) ) ;
#19373=DIRECTION ( 'NONE',  ( 4.147566128926370535E-16, 1.000000000000000000, -0.000000000000000000 ) ) ;
#19388=CARTESIAN_POINT ( 'NONE',  ( 831.1634899080286232, 239.9999999999999147, -202.7499999999998295 ) ) ;
#19426=VECTOR ( 'NONE', #19847, 1000.000000000000000 ) ;
#19440=DIRECTION ( 'NONE',  ( -1.880165489482579047E-16, -1.000000000000000000, -0.000000000000000000 ) ) ;
#19509=CARTESIAN_POINT ( 'NONE',  ( 959.5497976682736407, 239.9999999999998863, -2132.806278688367456 ) ) ;
#19562=CARTESIAN_POINT ( 'NONE',  ( -858.8365100919713768, 260.0000000000002274, -199.9999999999881481 ) ) ;
#19570=AXIS2_PLACEMENT_3D ( 'NONE', #4101, #32272, #11713 ) ;
#19590=VERTEX_POINT ( 'NONE', #20705 ) ;
#19671=CIRCLE ( 'NONE', #6432, 2.749999999999808153 ) ;
#19686=CARTESIAN_POINT ( 'NONE',  ( -521.6730038022808458, 240.0000000000001705, 350.0000000000000000 ) ) ;
#19695=ADVANCED_FACE ( 'NONE', ( #37585 ), #6412, .F. ) ;
#19717=ORIENTED_EDGE ( 'NONE', *, *, #45675, .F. ) ;
#19761=LINE ( 'NONE', #40563, #41682 ) ;
#19770=CARTESIAN_POINT ( 'NONE',  ( 571.1634899080285095, 229.9999999999999432, -197.2499999999982947 ) ) ;
#19772=ORIENTED_EDGE ( 'NONE', *, *, #39475, .F. ) ;
#19797=CARTESIAN_POINT ( 'NONE',  ( 701.1634899080286232, 239.9999999999999432, -197.2499999999991758 ) ) ;
#19824=VERTEX_POINT ( 'NONE', #2940 ) ;
#19828=PLANE ( 'NONE',  #1782 ) ;
#19847=DIRECTION ( 'NONE',  ( 1.000000000000000000, -1.880165489482579047E-16, 0.000000000000000000 ) ) ;
#19868=CIRCLE ( 'NONE', #35326, 2.749999999999919176 ) ;
#19871=DIRECTION ( 'NONE',  ( -1.000000000000000000, 0.000000000000000000, 0.000000000000000000 ) ) ;
#19887=CARTESIAN_POINT ( 'NONE',  ( 521.6730038022808458, 199.9999999999999147, -122.7905160835442615 ) ) ;
#19959=FACE_BOUND ( 'NONE', #22056, .T. ) ;
#19974=FACE_OUTER_BOUND ( 'NONE', #1533, .T. ) ;
#19988=DIRECTION ( 'NONE',  ( -0.000000000000000000, -0.000000000000000000, 1.000000000000000000 ) ) ;
#19989=DIRECTION ( 'NONE',  ( 0.000000000000000000, 0.000000000000000000, 1.000000000000000000 ) ) ;
#20005=VERTEX_POINT ( 'NONE', #14495 ) ;
#20029=CARTESIAN_POINT ( 'NONE',  ( -919.9999999999993179, 219.9999999999998863, -360.0000000000000000 ) ) ;
#20051=ORIENTED_EDGE ( 'NONE', *, *, #37699, .T. ) ;
#20109=ORIENTED_EDGE ( 'NONE', *, *, #20182, .T. ) ;
#20181=DIRECTION ( 'NONE',  ( 1.000000000000000000, -4.147566128926363633E-16, 0.000000000000000000 ) ) ;
#20182=EDGE_CURVE ( 'NONE', #12556, #38643, #45335, .T. ) ;
#20245=FACE_OUTER_BOUND ( 'NONE', #29789, .T. ) ;
#20246=FACE_OUTER_BOUND ( 'NONE', #3556, .T. ) ;
#20314=VECTOR ( 'NONE', #12406, 1000.000000000000000 ) ;
#20317=CARTESIAN_POINT ( 'NONE',  ( -919.9999999999993179, 154.9999999999998863, 350.0000000000000000 ) ) ;
#20355=ORIENTED_EDGE ( 'NONE', *, *, #17957, .T. ) ;
#20366=DIRECTION ( 'NONE',  ( -1.000000000000000000, 0.000000000000000000, 0.000000000000000000 ) ) ;
#20368=CARTESIAN_POINT ( 'NONE',  ( 441.1634899080286232, 229.9999999999999716, -199.9999999999972431 ) ) ;
#20393=EDGE_LOOP ( 'NONE', ( #16598, #9559 ) ) ;
#20398=ORIENTED_EDGE ( 'NONE', *, *, #5139, .F. ) ;
#20416=CARTESIAN_POINT ( 'NONE',  ( 454.7528517110262101, 239.9999999999999716, 350.0000000000000000 ) ) ;
#20423=VECTOR ( 'NONE', #15875, 1000.000000000000000 ) ;
#20433=VECTOR ( 'NONE', #23115, 1000.000000000000000 ) ;
#20494=DIRECTION ( 'NONE',  ( -0.000000000000000000, -0.000000000000000000, 1.000000000000000000 ) ) ;
#20504=DIRECTION ( 'NONE',  ( -0.000000000000000000, 0.000000000000000000, -1.000000000000000000 ) ) ;
#20516=VERTEX_POINT ( 'NONE', #33175 ) ;
#20529=CARTESIAN_POINT ( 'NONE',  ( 959.5497976682736407, 229.9999999999998579, -209.9999999999999716 ) ) ;
#20531=CYLINDRICAL_SURFACE ( 'NONE', #41105, 8.024999999999948841 ) ;
#20576=ORIENTED_EDGE ( 'NONE', *, *, #41103, .F. ) ;
#20579=LINE ( 'NONE', #45541, #41081 ) ;
#20584=CARTESIAN_POINT ( 'NONE',  ( 571.1634899080285095, 239.9999999999999716, -202.7499999999980105 ) ) ;
#20607=DIRECTION ( 'NONE',  ( 0.000000000000000000, 0.000000000000000000, 1.000000000000000000 ) ) ;
#20625=ORIENTED_EDGE ( 'NONE', *, *, #45596, .T. ) ;
#20629=DIRECTION ( 'NONE',  ( 1.880165489482579047E-16, 1.000000000000000000, 0.000000000000000000 ) ) ;
#20702=CARTESIAN_POINT ( 'NONE',  ( -454.7528517110260964, 200.0000000000001137, -122.7905160835438068 ) ) ;
#20705=CARTESIAN_POINT ( 'NONE',  ( 571.1634899080285095, 239.9999999999999716, -197.2499999999982947 ) ) ;
#20716=ORIENTED_EDGE ( 'NONE', *, *, #17129, .F. ) ;
#20739=EDGE_CURVE ( 'NONE', #10345, #9331, #27830, .T. ) ;
#20746=CARTESIAN_POINT ( 'NONE',  ( -728.8365100919714905, 230.0000000000001705, -197.2499999999891998 ) ) ;
#20837=ORIENTED_EDGE ( 'NONE', *, *, #37974, .F. ) ;
#20839=VERTEX_POINT ( 'NONE', #34747 ) ;
#20852=ORIENTED_EDGE ( 'NONE', *, *, #17049, .T. ) ;
#20856=VERTEX_POINT ( 'NONE', #34530 ) ;
#20870=DIRECTION ( 'NONE',  ( -1.880165489482579047E-16, -1.000000000000000000, -0.000000000000000000 ) ) ;
#20883=STYLED_ITEM('',(#45744),#32965);
#20893=ORIENTED_EDGE ( 'NONE', *, *, #31178, .F. ) ;
#20903=AXIS2_PLACEMENT_3D ( 'NONE', #22386, #43647, #40641 ) ;
#20934=CIRCLE ( 'NONE', #23124, 2.749999999999842792 ) ;
#20943=ORIENTED_EDGE ( 'NONE', *, *, #35323, .F. ) ;
#20964=CIRCLE ( 'NONE', #1067, 2.749999999999919176 ) ;
#21010=VERTEX_POINT ( 'NONE', #14669 ) ;
#21040=CIRCLE ( 'NONE', #31361, 2.749999999999919176 ) ;
#21050=EDGE_CURVE ( 'NONE', #9329, #12718, #28263, .T. ) ;
#21074=ORIENTED_EDGE ( 'NONE', *, *, #25004, .T. ) ;
#21126=CIRCLE ( 'NONE', #10809, 8.024999999999948841 ) ;
#21165=FACE_OUTER_BOUND ( 'NONE', #42784, .T. ) ;
#21176=FACE_OUTER_BOUND ( 'NONE', #228, .T. ) ;
#21212=LINE ( 'NONE', #11054, #40828 ) ;
#21228=AXIS2_PLACEMENT_3D ( 'NONE', #29156, #24997, #39108 ) ;
#21247=EDGE_LOOP ( 'NONE', ( #44263, #13713, #14949, #28418 ) ) ;
#21264=VERTEX_POINT ( 'NONE', #17890 ) ;
#21266=FACE_OUTER_BOUND ( 'NONE', #34841, .T. ) ;
#21314=ORIENTED_EDGE ( 'NONE', *, *, #35945, .F. ) ;
#21322=VECTOR ( 'NONE', #19871, 1000.000000000000000 ) ;
#21362=ORIENTED_EDGE ( 'NONE', *, *, #426, .T. ) ;
#21438=DIRECTION ( 'NONE',  ( 1.000000000000000000, 0.000000000000000000, 0.000000000000000000 ) ) ;
#21462=DIRECTION ( 'NONE',  ( 1.000000000000000000, 0.000000000000000000, 0.000000000000000000 ) ) ;
#21512=ADVANCED_FACE ( 'NONE', ( #22919 ), #4933, .F. ) ;
#21517=ADVANCED_FACE ( 'NONE', ( #29637, #26399, #8181, #18580, #15775, #1902, #40500, #22246, #37010, #8638, #32663, #7967, #22700, #36343, #16011 ), #12326, .T. ) ;
#21534=EDGE_LOOP ( 'NONE', ( #40580, #6823 ) ) ;
#21549=DIRECTION ( 'NONE',  ( 1.000000000000000000, 0.000000000000000000, 0.000000000000000000 ) ) ;
#21610=AXIS2_PLACEMENT_3D ( 'NONE', #28089, #10315, #42651 ) ;
#21613=DIRECTION ( 'NONE',  ( -0.000000000000000000, -0.000000000000000000, 1.000000000000000000 ) ) ;
#21633=LINE ( 'NONE', #35715, #30152 ) ;
#21655=VECTOR ( 'NONE', #5679, 1000.000000000000000 ) ;
#21679=CARTESIAN_POINT ( 'NONE',  ( -959.5497976682736407, 240.0000000000002274, -2132.806278688367456 ) ) ;
#21743=LINE ( 'NONE', #28689, #39501 ) ;
#21745=AXIS2_PLACEMENT_3D ( 'NONE', #9004, #33487, #36734 ) ;
#21777=CIRCLE ( 'NONE', #1843, 2.749999999999919176 ) ;
#21779=CARTESIAN_POINT ( 'NONE',  ( -454.7528517110260964, 240.0000000000001421, -122.7905160835438068 ) ) ;
#21780=CARTESIAN_POINT ( 'NONE',  ( 521.6730038022808458, 239.9999999999999432, -122.7905160835442615 ) ) ;
#21793=CARTESIAN_POINT ( 'NONE',  ( 181.1634899080285948, 240.0000000000000284, -197.2499999999955662 ) ) ;
#21796=DIRECTION ( 'NONE',  ( -0.000000000000000000, 1.000000000000000000, -0.000000000000000000 ) ) ;
#21824=EDGE_CURVE ( 'NONE', #19590, #19031, #45376, .T. ) ;
#21855=EDGE_CURVE ( 'NONE', #24181, #32406, #40349, .T. ) ;
#21856=DIRECTION ( 'NONE',  ( 0.000000000000000000, 0.000000000000000000, 1.000000000000000000 ) ) ;
#21878=( NAMED_UNIT ( * ) SI_UNIT ( $, .STERADIAN. ) SOLID_ANGLE_UNIT ( ) );
#21885=AXIS2_PLACEMENT_3D ( 'NONE', #35633, #308, #22621 ) ;
#21886=EDGE_CURVE ( 'NONE', #7811, #20516, #19761, .T. ) ;
#21897=EDGE_CURVE ( 'NONE', #26734, #33702, #16293, .T. ) ;
#21901=ADVANCED_FACE ( 'NONE', ( #12824 ), #26905, .F. ) ;
#21909=LINE ( 'NONE', #25813, #24079 ) ;
#21920=DIRECTION ( 'NONE',  ( 1.000000000000000000, 0.000000000000000000, 0.000000000000000000 ) ) ;
#21937=AXIS2_PLACEMENT_3D ( 'NONE', #43091, #4072, #39653 ) ;
#21943=ORIENTED_EDGE ( 'NONE', *, *, #22712, .T. ) ;
#21964=DIRECTION ( 'NONE',  ( 1.000000000000000000, 0.000000000000000000, 0.000000000000000000 ) ) ;
#21967=ORIENTED_EDGE ( 'NONE', *, *, #15575, .T. ) ;
#22008=VERTEX_POINT ( 'NONE', #24126 ) ;
#22028=CARTESIAN_POINT ( 'NONE',  ( -78.83651009197140525, 260.0000000000000568, -197.2499999999937756 ) ) ;
#22035=ORIENTED_EDGE ( 'NONE', *, *, #22712, .F. ) ;
#22052=CIRCLE ( 'NONE', #22766, 2.749999999999863665 ) ;
#22056=EDGE_LOOP ( 'NONE', ( #28594, #29289 ) ) ;
#22081=CARTESIAN_POINT ( 'NONE',  ( 571.1634899080285095, 259.9999999999999432, -199.9999999999981526 ) ) ;
#22119=DIRECTION ( 'NONE',  ( 1.000000000000000000, -1.880165489482579047E-16, 0.000000000000000000 ) ) ;
#22124=CARTESIAN_POINT ( 'NONE',  ( 959.5497976682736407, 120.6654763175833693, -209.9999999999999716 ) ) ;
#22128=FACE_OUTER_BOUND ( 'NONE', #8151, .T. ) ;
#22171=LINE ( 'NONE', #40193, #32183 ) ;
#22194=FACE_OUTER_BOUND ( 'NONE', #34137, .T. ) ;
#22214=ORIENTED_EDGE ( 'NONE', *, *, #26932, .T. ) ;
#22226=CARTESIAN_POINT ( 'NONE',  ( 51.16348990802859475, 240.0000000000000568, -202.7499999999943441 ) ) ;
#22229=EDGE_LOOP ( 'NONE', ( #17177, #41581, #19717, #4408, #25103, #42498, #36927, #13384, #12970, #6093, #29278, #23616 ) ) ;
#22246=FACE_BOUND ( 'NONE', #36587, .T. ) ;
#22252=DIRECTION ( 'NONE',  ( -1.880165489482579047E-16, -1.000000000000000000, -0.000000000000000000 ) ) ;
#22269=ORIENTED_EDGE ( 'NONE', *, *, #32364, .F. ) ;
#22278=CARTESIAN_POINT ( 'NONE',  ( -598.8365100919716042, 230.0000000000001421, -197.2499999999901092 ) ) ;
#22285=CARTESIAN_POINT ( 'NONE',  ( -728.8365100919714905, 260.0000000000001705, -199.9999999999890861 ) ) ;
#22286=LINE ( 'NONE', #1283, #40295 ) ;
#22314=EDGE_LOOP ( 'NONE', ( #4901, #26632, #35334, #17867 ) ) ;
#22330=FACE_BOUND ( 'NONE', #5229, .T. ) ;
#22351=CIRCLE ( 'NONE', #15735, 2.749999999999808153 ) ;
#22356=DIRECTION ( 'NONE',  ( -0.000000000000000000, 1.000000000000000000, -0.000000000000000000 ) ) ;
#22369=CARTESIAN_POINT ( 'NONE',  ( -949.5497976682736407, 120.6654763175833693, -209.9999999999999716 ) ) ;
#22370=ORIENTED_EDGE ( 'NONE', *, *, #45621, .T. ) ;
#22386=CARTESIAN_POINT ( 'NONE',  ( 311.1634899080286232, 260.0000000000000000, -199.9999999999963336 ) ) ;
#22409=DIRECTION ( 'NONE',  ( 0.000000000000000000, 0.000000000000000000, 1.000000000000000000 ) ) ;
#22446=DIRECTION ( 'NONE',  ( -0.000000000000000000, 1.000000000000000000, 0.000000000000000000 ) ) ;
#22447=FACE_BOUND ( 'NONE', #40169, .T. ) ;
#22449=AXIS2_PLACEMENT_3D ( 'NONE', #5156, #11414, #19240 ) ;
#22475=LINE ( 'NONE', #26176, #10717 ) ;
#22489=EDGE_CURVE ( 'NONE', #24672, #13253, #30627, .T. ) ;
#22492=DIRECTION ( 'NONE',  ( 1.000000000000000000, 0.000000000000000000, 0.000000000000000000 ) ) ;
#22519=VECTOR ( 'NONE', #32773, 1000.000000000000000 ) ;
#22544=CARTESIAN_POINT ( 'NONE',  ( -598.8365100919716042, 260.0000000000001705, -199.9999999999899671 ) ) ;
#22575=VECTOR ( 'NONE', #17289, 1000.000000000000000 ) ;
#22591=EDGE_LOOP ( 'NONE', ( #27916, #22888, #41951, #6375 ) ) ;
#22621=DIRECTION ( 'NONE',  ( 1.000000000000000000, 0.000000000000000000, 0.000000000000000000 ) ) ;
#22642=DIRECTION ( 'NONE',  ( 1.000000000000000000, -1.880165489482579047E-16, -0.000000000000000000 ) ) ;
#22696=EDGE_CURVE ( 'NONE', #928, #282, #29894, .T. ) ;
#22700=FACE_BOUND ( 'NONE', #26050, .T. ) ;
#22712=EDGE_CURVE ( 'NONE', #43744, #1441, #22475, .T. ) ;
#22722=( NAMED_UNIT ( * ) PLANE_ANGLE_UNIT ( ) SI_UNIT ( $, .RADIAN. ) );
#22729=AXIS2_PLACEMENT_3D ( 'NONE', #19887, #34429, #3241 ) ;
#22748=DIRECTION ( 'NONE',  ( -1.880165489482579047E-16, -1.000000000000000000, -0.000000000000000000 ) ) ;
#22766=AXIS2_PLACEMENT_3D ( 'NONE', #16918, #37475, #13230 ) ;
#22784=EDGE_LOOP ( 'NONE', ( #7350, #23574, #32399, #13809 ) ) ;
#22831=FACE_OUTER_BOUND ( 'NONE', #29095, .T. ) ;
#22838=APPLICATION_CONTEXT ( 'automotive_design' ) ;
#22888=ORIENTED_EDGE ( 'NONE', *, *, #7510, .T. ) ;
#22912=CARTESIAN_POINT ( 'NONE',  ( 959.5497976682736407, 239.9999999999998863, 350.0000000000000000 ) ) ;
#22919=FACE_OUTER_BOUND ( 'NONE', #8978, .T. ) ;
#22924=DIRECTION ( 'NONE',  ( 0.000000000000000000, -1.000000000000000000, 0.000000000000000000 ) ) ;
#22940=ORIENTED_EDGE ( 'NONE', *, *, #22696, .T. ) ;
#22962=EDGE_CURVE ( 'NONE', #26734, #32683, #34926, .T. ) ;
#22981=EDGE_CURVE ( 'NONE', #34173, #22008, #30543, .T. ) ;
#23016=EDGE_CURVE ( 'NONE', #33397, #9428, #10441, .T. ) ;
#23028=VERTEX_POINT ( 'NONE', #24516 ) ;
#23033=FACE_OUTER_BOUND ( 'NONE', #36718, .T. ) ;
#23035=ORIENTED_EDGE ( 'NONE', *, *, #42173, .F. ) ;
#23058=VERTEX_POINT ( 'NONE', #41874 ) ;
#23069=PRODUCT_DEFINITION_FORMATION_WITH_SPECIFIED_SOURCE ( 'ANY', '', #2245, .NOT_KNOWN. ) ;
#23115=DIRECTION ( 'NONE',  ( -0.000000000000000000, 1.000000000000000000, -0.000000000000000000 ) ) ;
#23124=AXIS2_PLACEMENT_3D ( 'NONE', #4754, #29471, #25772 ) ;
#23149=EDGE_CURVE ( 'NONE', #24787, #19824, #27095, .T. ) ;
#23153=CARTESIAN_POINT ( 'NONE',  ( 0.000000000000000000, 0.000000000000000000, 0.000000000000000000 ) ) ;
#23167=DIRECTION ( 'NONE',  ( -0.000000000000000000, 1.000000000000000000, -0.000000000000000000 ) ) ;
#23208=AXIS2_PLACEMENT_3D ( 'NONE', #25874, #8570, #37173 ) ;
#23261=VERTEX_POINT ( 'NONE', #42170 ) ;
#23357=FACE_OUTER_BOUND ( 'NONE', #39158, .T. ) ;
#23386=ORIENTED_EDGE ( 'NONE', *, *, #43860, .T. ) ;
#23405=AXIS2_PLACEMENT_3D ( 'NONE', #35251, #31779, #38727 ) ;
#23409=ORIENTED_EDGE ( 'NONE', *, *, #20739, .F. ) ;
#23416=CIRCLE ( 'NONE', #21228, 8.024999999999948841 ) ;
#23439=DIRECTION ( 'NONE',  ( 1.880165489482579047E-16, 1.000000000000000000, -0.000000000000000000 ) ) ;
#23440=DIRECTION ( 'NONE',  ( 1.000000000000000000, 0.000000000000000000, 0.000000000000000000 ) ) ;
#23447=LINE ( 'NONE', #26246, #21655 ) ;
#23449=ORIENTED_EDGE ( 'NONE', *, *, #4417, .F. ) ;
#23474=CARTESIAN_POINT ( 'NONE',  ( -949.5497976682736407, 240.0000000000002274, 339.9999999999998863 ) ) ;
#23493=LINE ( 'NONE', #41300, #24677 ) ;
#23495=ORIENTED_EDGE ( 'NONE', *, *, #16791, .T. ) ;
#23498=CARTESIAN_POINT ( 'NONE',  ( 959.5497976682736407, 229.9999999999998579, -122.7905160835440768 ) ) ;
#23519=LINE ( 'NONE', #33927, #35133 ) ;
#23535=EDGE_CURVE ( 'NONE', #39949, #30067, #41016, .T. ) ;
#23538=CARTESIAN_POINT ( 'NONE',  ( -728.8365100919714905, 240.0000000000001990, -199.9999999999890861 ) ) ;
#23574=ORIENTED_EDGE ( 'NONE', *, *, #37138, .T. ) ;
#23604=DIRECTION ( 'NONE',  ( -0.000000000000000000, -0.000000000000000000, 1.000000000000000000 ) ) ;
#23607=ORIENTED_EDGE ( 'NONE', *, *, #43619, .T. ) ;
#23613=CARTESIAN_POINT ( 'NONE',  ( 831.1634899080286232, 259.9999999999998863, -199.9999999999999432 ) ) ;
#23616=ORIENTED_EDGE ( 'NONE', *, *, #640, .F. ) ;
#23685=DIRECTION ( 'NONE',  ( -0.000000000000000000, 1.000000000000000000, -0.000000000000000000 ) ) ;
#23719=CARTESIAN_POINT ( 'NONE',  ( 8.295132257852746908E-14, 200.0000000000001421, 350.0000000000000000 ) ) ;
#23819=DIRECTION ( 'NONE',  ( -0.000000000000000000, 1.000000000000000000, 0.000000000000000000 ) ) ;
#23860=AXIS2_PLACEMENT_3D ( 'NONE', #16973, #20870, #95 ) ;
#23897=DIRECTION ( 'NONE',  ( -1.880165489482579047E-16, -1.000000000000000000, -0.000000000000000000 ) ) ;
#23920=DIRECTION ( 'NONE',  ( -0.000000000000000000, 1.000000000000000000, -0.000000000000000000 ) ) ;
#23932=AXIS2_PLACEMENT_3D ( 'NONE', #33993, #33779, #43940 ) ;
#23949=VECTOR ( 'NONE', #28194, 1000.000000000000000 ) ;
#23962=VECTOR ( 'NONE', #22642, 1000.000000000000000 ) ;
#23972=CIRCLE ( 'NONE', #19570, 2.749999999999919176 ) ;
#24043=AXIS2_PLACEMENT_3D ( 'NONE', #31875, #6322, #27119 ) ;
#24071=VERTEX_POINT ( 'NONE', #16038 ) ;
#24074=EDGE_LOOP ( 'NONE', ( #20943, #28596, #24777, #40608 ) ) ;
#24079=VECTOR ( 'NONE', #32059, 1000.000000000000000 ) ;
#24126=CARTESIAN_POINT ( 'NONE',  ( -521.6730038022808458, 200.0000000000001421, 350.0000000000000000 ) ) ;
#24134=DIRECTION ( 'NONE',  ( -0.000000000000000000, 1.000000000000000000, -0.000000000000000000 ) ) ;
#24148=AXIS2_PLACEMENT_3D ( 'NONE', #35668, #11203, #39164 ) ;
#24163=CARTESIAN_POINT ( 'NONE',  ( -78.83651009197140525, 260.0000000000000568, -199.9999999999936051 ) ) ;
#24168=DIRECTION ( 'NONE',  ( -0.000000000000000000, -0.000000000000000000, 1.000000000000000000 ) ) ;
#24169=FACE_OUTER_BOUND ( 'NONE', #12388, .T. ) ;
#24181=VERTEX_POINT ( 'NONE', #3943 ) ;
#24220=ORIENTED_EDGE ( 'NONE', *, *, #22962, .F. ) ;
#24230=CARTESIAN_POINT ( 'NONE',  ( -208.8365100919714052, 230.0000000000000853, -202.7499999999925251 ) ) ;
#24281=DIRECTION ( 'NONE',  ( -1.880165489482579047E-16, -1.000000000000000000, -0.000000000000000000 ) ) ;
#24287=ADVANCED_FACE ( 'NONE', ( #21266 ), #17584, .F. ) ;
#24376=ORIENTED_EDGE ( 'NONE', *, *, #25533, .T. ) ;
#24407=VERTEX_POINT ( 'NONE', #1385 ) ;
#24430=DIRECTION ( 'NONE',  ( -1.880165489482579047E-16, -1.000000000000000000, -0.000000000000000000 ) ) ;
#24467=ORIENTED_EDGE ( 'NONE', *, *, #32624, .T. ) ;
#24473=CARTESIAN_POINT ( 'NONE',  ( -949.5497976682736407, 120.6654763175833693, 339.9999999999999432 ) ) ;
#24516=CARTESIAN_POINT ( 'NONE',  ( -78.83651009197140525, 230.0000000000000568, -197.2499999999937756 ) ) ;
#24540=CARTESIAN_POINT ( 'NONE',  ( -521.6730038022808458, 9.808315785437627339E-14, 350.0000000000000000 ) ) ;
#24541=FACE_OUTER_BOUND ( 'NONE', #17769, .T. ) ;
#24549=LINE ( 'NONE', #41675, #43090 ) ;
#24575=EDGE_LOOP ( 'NONE', ( #43243, #1042 ) ) ;
#24615=CARTESIAN_POINT ( 'NONE',  ( -208.8365100919714052, 240.0000000000001137, -197.2499999999928377 ) ) ;
#24631=FACE_OUTER_BOUND ( 'NONE', #36912, .T. ) ;
#24640=EDGE_CURVE ( 'NONE', #791, #282, #22171, .T. ) ;
#24641=AXIS2_PLACEMENT_3D ( 'NONE', #25622, #22356, #18254 ) ;
#24660=LINE ( 'NONE', #42229, #26041 ) ;
#24672=VERTEX_POINT ( 'NONE', #18284 ) ;
#24677=VECTOR ( 'NONE', #16121, 1000.000000000000000 ) ;
#24688=FACE_BOUND ( 'NONE', #1872, .T. ) ;
#24712=VECTOR ( 'NONE', #2837, 1000.000000000000000 ) ;
#24744=DIRECTION ( 'NONE',  ( 1.000000000000000000, 0.000000000000000000, 0.000000000000000000 ) ) ;
#24766=AXIS2_PLACEMENT_3D ( 'NONE', #18561, #28947, #36780 ) ;
#24769=LINE ( 'NONE', #25688, #25648 ) ;
#24772=VECTOR ( 'NONE', #9567, 1000.000000000000000 ) ;
#24777=ORIENTED_EDGE ( 'NONE', *, *, #21050, .T. ) ;
#24782=AXIS2_PLACEMENT_3D ( 'NONE', #32784, #11989, #7230 ) ;
#24787=VERTEX_POINT ( 'NONE', #34139 ) ;
#24871=AXIS2_PLACEMENT_3D ( 'NONE', #18678, #44452, #37293 ) ;
#24939=ORIENTED_EDGE ( 'NONE', *, *, #7143, .T. ) ;
#24942=AXIS2_PLACEMENT_3D ( 'NONE', #30664, #17499, #31577 ) ;
#24976=DIRECTION ( 'NONE',  ( -1.880165489482579047E-16, -1.000000000000000000, -0.000000000000000000 ) ) ;
#24997=DIRECTION ( 'NONE',  ( -0.000000000000000000, -0.000000000000000000, -1.000000000000000000 ) ) ;
#25004=EDGE_CURVE ( 'NONE', #15202, #10227, #23519, .T. ) ;
#25103=ORIENTED_EDGE ( 'NONE', *, *, #39979, .T. ) ;
#25108=ORIENTED_EDGE ( 'NONE', *, *, #30616, .T. ) ;
#25131=EDGE_LOOP ( 'NONE', ( #17690, #31652, #23607, #31438 ) ) ;
#25210=EDGE_CURVE ( 'NONE', #5848, #43744, #3198, .T. ) ;
#25265=CARTESIAN_POINT ( 'NONE',  ( 701.1634899080286232, 229.9999999999999147, -199.9999999999990337 ) ) ;
#25306=DIRECTION ( 'NONE',  ( 1.880165489482579047E-16, 1.000000000000000000, 0.000000000000000000 ) ) ;
#25319=CYLINDRICAL_SURFACE ( 'NONE', #15404, 2.749999999999835687 ) ;
#25327=ORIENTED_EDGE ( 'NONE', *, *, #640, .T. ) ;
#25397=ORIENTED_EDGE ( 'NONE', *, *, #1807, .T. ) ;
#25405=ORIENTED_EDGE ( 'NONE', *, *, #31393, .T. ) ;
#25444=AXIS2_PLACEMENT_3D ( 'NONE', #28108, #20504, #34593 ) ;
#25471=DIRECTION ( 'NONE',  ( -1.000000000000000000, 4.147566128926363633E-16, 0.000000000000000000 ) ) ;
#25483=DIRECTION ( 'NONE',  ( 1.000000000000000000, 0.000000000000000000, 0.000000000000000000 ) ) ;
#25486=AXIS2_PLACEMENT_3D ( 'NONE', #25265, #4493, #18585 ) ;
#25504=VECTOR ( 'NONE', #28776, 1000.000000000000000 ) ;
#25506=CARTESIAN_POINT ( 'NONE',  ( -728.8365100919714905, 240.0000000000001990, -199.9999999999890861 ) ) ;
#25533=EDGE_CURVE ( 'NONE', #12108, #45635, #18904, .T. ) ;
#25540=CYLINDRICAL_SURFACE ( 'NONE', #36664, 2.749999999999835687 ) ;
#25545=CARTESIAN_POINT ( 'NONE',  ( -454.7528517110260964, 200.0000000000001137, -122.7905160835438068 ) ) ;
#25605=DIRECTION ( 'NONE',  ( -0.000000000000000000, -0.000000000000000000, -1.000000000000000000 ) ) ;
#25622=CARTESIAN_POINT ( 'NONE',  ( 441.1634899080286232, 259.9999999999999432, -199.9999999999972431 ) ) ;
#25648=VECTOR ( 'NONE', #15069, 1000.000000000000000 ) ;
#25688=CARTESIAN_POINT ( 'NONE',  ( -928.0249999999991815, 154.9999999999998863, -360.0000000000000000 ) ) ;
#25708=ORIENTED_EDGE ( 'NONE', *, *, #36696, .T. ) ;
#25726=DIRECTION ( 'NONE',  ( -0.000000000000000000, 1.000000000000000000, -0.000000000000000000 ) ) ;
#25743=CIRCLE ( 'NONE', #11019, 8.024999999999948841 ) ;
#25747=EDGE_CURVE ( 'NONE', #17477, #928, #21909, .T. ) ;
#25763=DIRECTION ( 'NONE',  ( -0.000000000000000000, 1.000000000000000000, -0.000000000000000000 ) ) ;
#25772=DIRECTION ( 'NONE',  ( 1.000000000000000000, 0.000000000000000000, 0.000000000000000000 ) ) ;
#25809=FACE_BOUND ( 'NONE', #16881, .T. ) ;
#25811=EDGE_CURVE ( 'NONE', #28460, #13538, #42692, .T. ) ;
#25813=CARTESIAN_POINT ( 'NONE',  ( 911.9749999999993406, 219.9999999999998863, -360.0000000000000000 ) ) ;
#25821=ORIENTED_EDGE ( 'NONE', *, *, #43619, .F. ) ;
#25849=EDGE_CURVE ( 'NONE', #23261, #35455, #7590, .T. ) ;
#25852=ORIENTED_EDGE ( 'NONE', *, *, #27824, .F. ) ;
#25874=CARTESIAN_POINT ( 'NONE',  ( 441.1634899080286232, 240.0000000000000000, -199.9999999999972431 ) ) ;
#25899=DIRECTION ( 'NONE',  ( -0.000000000000000000, 1.000000000000000000, -0.000000000000000000 ) ) ;
#25907=ORIENTED_EDGE ( 'NONE', *, *, #40496, .T. ) ;
#25918=CARTESIAN_POINT ( 'NONE',  ( -521.6730038022808458, 9.808315785437627339E-14, 339.9999999999999432 ) ) ;
#25951=ORIENTED_EDGE ( 'NONE', *, *, #27454, .F. ) ;
#25958=VECTOR ( 'NONE', #28788, 1000.000000000000000 ) ;
#25960=ORIENTED_EDGE ( 'NONE', *, *, #13763, .F. ) ;
#25967=ORIENTED_EDGE ( 'NONE', *, *, #26932, .F. ) ;
#25989=CARTESIAN_POINT ( 'NONE',  ( 521.6730038022808458, 239.9999999999999432, 350.0000000000000000 ) ) ;
#26007=AXIS2_PLACEMENT_3D ( 'NONE', #38491, #378, #3397 ) ;
#26009=EDGE_LOOP ( 'NONE', ( #36547, #26126 ) ) ;
#26030=CARTESIAN_POINT ( 'NONE',  ( -208.8365100919714052, 260.0000000000001137, -199.9999999999926956 ) ) ;
#26041=VECTOR ( 'NONE', #10582, 1000.000000000000000 ) ;
#26050=EDGE_LOOP ( 'NONE', ( #9382, #11848 ) ) ;
#26058=EDGE_CURVE ( 'NONE', #10523, #17262, #44783, .T. ) ;
#26126=ORIENTED_EDGE ( 'NONE', *, *, #26058, .F. ) ;
#26129=CIRCLE ( 'NONE', #41634, 2.749999999999863665 ) ;
#26130=ORIENTED_EDGE ( 'NONE', *, *, #14615, .T. ) ;
#26149=CARTESIAN_POINT ( 'NONE',  ( 911.9749999999993406, 154.9999999999998863, -360.0000000000000000 ) ) ;
#26150=ORIENTED_EDGE ( 'NONE', *, *, #28627, .F. ) ;
#26172=EDGE_LOOP ( 'NONE', ( #34678, #14684, #40176, #9663 ) ) ;
#26176=CARTESIAN_POINT ( 'NONE',  ( 949.5497976682736407, 239.9999999999998863, -209.9999999999999716 ) ) ;
#26179=EDGE_LOOP ( 'NONE', ( #42099, #32972, #29501, #20051, #17966, #11563 ) ) ;
#26187=ORIENTED_EDGE ( 'NONE', *, *, #402, .F. ) ;
#26246=CARTESIAN_POINT ( 'NONE',  ( -858.8365100919713768, 260.0000000000002274, -202.7499999999880345 ) ) ;
#26269=DIRECTION ( 'NONE',  ( -1.000000000000000000, 0.000000000000000000, 0.000000000000000000 ) ) ;
#26383=ADVANCED_FACE ( 'NONE', ( #21165 ), #3392, .F. ) ;
#26388=CARTESIAN_POINT ( 'NONE',  ( 701.1634899080286232, 239.9999999999999432, -199.9999999999990337 ) ) ;
#26399=FACE_BOUND ( 'NONE', #26009, .T. ) ;
#26425=ORIENTED_EDGE ( 'NONE', *, *, #4111, .T. ) ;
#26493=CARTESIAN_POINT ( 'NONE',  ( 959.5497976682736407, 120.6654763175833693, 339.9999999999998863 ) ) ;
#26497=CYLINDRICAL_SURFACE ( 'NONE', #4228, 2.749999999999863665 ) ;
#26615=AXIS2_PLACEMENT_3D ( 'NONE', #26388, #8627, #12742 ) ;
#26631=ADVANCED_FACE ( 'NONE', ( #7538 ), #4523, .F. ) ;
#26632=ORIENTED_EDGE ( 'NONE', *, *, #7420, .T. ) ;
#26633=FACE_OUTER_BOUND ( 'NONE', #1127, .T. ) ;
#26636=EDGE_CURVE ( 'NONE', #15138, #27605, #18171, .T. ) ;
#26639=ORIENTED_EDGE ( 'NONE', *, *, #43810, .F. ) ;
#26649=AXIS2_PLACEMENT_3D ( 'NONE', #12526, #5591, #1661 ) ;
#26653=ADVANCED_FACE ( 'NONE', ( #18396 ), #3840, .F. ) ;
#26716=DIRECTION ( 'NONE',  ( 0.000000000000000000, 0.000000000000000000, -1.000000000000000000 ) ) ;
#26718=ADVANCED_FACE ( 'NONE', ( #11456 ), #25540, .F. ) ;
#26734=VERTEX_POINT ( 'NONE', #15382 ) ;
#26755=ORIENTED_EDGE ( 'NONE', *, *, #25004, .F. ) ;
#26759=DIRECTION ( 'NONE',  ( 1.000000000000000000, -1.880165489482579047E-16, 0.000000000000000000 ) ) ;
#26780=AXIS2_PLACEMENT_3D ( 'NONE', #22544, #39685, #36412 ) ;
#26822=CARTESIAN_POINT ( 'NONE',  ( -858.8365100919713768, 240.0000000000002274, -199.9999999999881481 ) ) ;
#26853=ORIENTED_EDGE ( 'NONE', *, *, #17668, .F. ) ;
#26858=AXIS2_PLACEMENT_3D ( 'NONE', #23153, #34241, #6075 ) ;
#26870=ORIENTED_EDGE ( 'NONE', *, *, #42492, .F. ) ;
#26878=AXIS2_PLACEMENT_3D ( 'NONE', #27425, #6422, #37826 ) ;
#26884=CARTESIAN_POINT ( 'NONE',  ( -959.5497976682736407, 240.0000000000002274, 350.0000000000000000 ) ) ;
#26892=DIRECTION ( 'NONE',  ( -1.880165489482579047E-16, -1.000000000000000000, 0.000000000000000000 ) ) ;
#26905=CYLINDRICAL_SURFACE ( 'NONE', #31350, 8.024999999999948841 ) ;
#26932=EDGE_CURVE ( 'NONE', #1769, #42109, #11228, .T. ) ;
#26965=ORIENTED_EDGE ( 'NONE', *, *, #45245, .T. ) ;
#27000=EDGE_LOOP ( 'NONE', ( #6431, #26965, #30666, #11925 ) ) ;
#27055=VECTOR ( 'NONE', #18907, 1000.000000000000000 ) ;
#27072=LINE ( 'NONE', #37219, #28539 ) ;
#27086=VECTOR ( 'NONE', #32532, 1000.000000000000000 ) ;
#27095=LINE ( 'NONE', #16702, #33587 ) ;
#27108=ORIENTED_EDGE ( 'NONE', *, *, #45675, .T. ) ;
#27109=CYLINDRICAL_SURFACE ( 'NONE', #34985, 2.749999999999835687 ) ;
#27119=DIRECTION ( 'NONE',  ( 0.000000000000000000, 0.000000000000000000, 1.000000000000000000 ) ) ;
#27188=CARTESIAN_POINT ( 'NONE',  ( -858.8365100919713768, 230.0000000000001990, -202.7499999999880345 ) ) ;
#27328=ORIENTED_EDGE ( 'NONE', *, *, #38163, .T. ) ;
#27330=VERTEX_POINT ( 'NONE', #10474 ) ;
#27331=DIRECTION ( 'NONE',  ( -1.880165489482579047E-16, -1.000000000000000000, -0.000000000000000000 ) ) ;
#27334=ORIENTED_EDGE ( 'NONE', *, *, #33712, .T. ) ;
#27341=CARTESIAN_POINT ( 'NONE',  ( 181.1634899080285948, 230.0000000000000000, -199.9999999999953957 ) ) ;
#27366=DIRECTION ( 'NONE',  ( -0.000000000000000000, 1.000000000000000000, -0.000000000000000000 ) ) ;
#27381=VERTEX_POINT ( 'NONE', #20416 ) ;
#27395=DIRECTION ( 'NONE',  ( -0.000000000000000000, 1.000000000000000000, -0.000000000000000000 ) ) ;
#27407=CARTESIAN_POINT ( 'NONE',  ( 521.6730038022808458, 199.9999999999999147, 339.9999999999999432 ) ) ;
#27425=CARTESIAN_POINT ( 'NONE',  ( 919.9999999999993179, 154.9999999999998863, 350.0000000000000000 ) ) ;
#27452=FACE_OUTER_BOUND ( 'NONE', #27900, .T. ) ;
#27454=EDGE_CURVE ( 'NONE', #1441, #23261, #24549, .T. ) ;
#27582=CARTESIAN_POINT ( 'NONE',  ( -858.8365100919713768, 240.0000000000002274, -202.7499999999880345 ) ) ;
#27585=AXIS2_PLACEMENT_3D ( 'NONE', #8169, #36110, #29182 ) ;
#27605=VERTEX_POINT ( 'NONE', #37746 ) ;
#27775=EDGE_CURVE ( 'NONE', #44488, #24071, #15039, .T. ) ;
#27788=VECTOR ( 'NONE', #26269, 1000.000000000000000 ) ;
#27798=EDGE_CURVE ( 'NONE', #14856, #24787, #14416, .T. ) ;
#27801=CARTESIAN_POINT ( 'NONE',  ( -454.7528517110261532, 8.550106180308601742E-14, 350.0000000000000000 ) ) ;
#27824=EDGE_CURVE ( 'NONE', #338, #33957, #43794, .T. ) ;
#27830=LINE ( 'NONE', #13751, #44574 ) ;
#27875=DIRECTION ( 'NONE',  ( 0.000000000000000000, 0.000000000000000000, 1.000000000000000000 ) ) ;
#27900=EDGE_LOOP ( 'NONE', ( #4503, #3503, #30812, #42746 ) ) ;
#27906=ORIENTED_EDGE ( 'NONE', *, *, #39475, .T. ) ;
#27913=CARTESIAN_POINT ( 'NONE',  ( -208.8365100919714052, 230.0000000000000853, -199.9999999999926956 ) ) ;
#27916=ORIENTED_EDGE ( 'NONE', *, *, #13757, .F. ) ;
#27995=CARTESIAN_POINT ( 'NONE',  ( -521.6730038022808458, 200.0000000000001421, -122.7905160835438068 ) ) ;
#28002=ADVANCED_FACE ( 'NONE', ( #32428 ), #777, .T. ) ;
#28007=ORIENTED_EDGE ( 'NONE', *, *, #21897, .T. ) ;
#28015=EDGE_LOOP ( 'NONE', ( #22035, #2762, #11168, #45339, #21362, #17914, #18949, #27328 ) ) ;
#28089=CARTESIAN_POINT ( 'NONE',  ( 51.16348990802859475, 230.0000000000000284, -199.9999999999945146 ) ) ;
#28108=CARTESIAN_POINT ( 'NONE',  ( 0.000000000000000000, 0.000000000000000000, 350.0000000000000000 ) ) ;
#28194=DIRECTION ( 'NONE',  ( -0.000000000000000000, 1.000000000000000000, -0.000000000000000000 ) ) ;
#28219=ORIENTED_EDGE ( 'NONE', *, *, #33989, .T. ) ;
#28246=DIRECTION ( 'NONE',  ( 1.000000000000000000, 0.000000000000000000, 0.000000000000000000 ) ) ;
#28263=LINE ( 'NONE', #42609, #1118 ) ;
#28295=DIRECTION ( 'NONE',  ( 0.000000000000000000, -1.000000000000000000, 0.000000000000000000 ) ) ;
#28304=DIRECTION ( 'NONE',  ( -1.880165489482579047E-16, -1.000000000000000000, -0.000000000000000000 ) ) ;
#28321=LINE ( 'NONE', #162, #10953 ) ;
#28409=ORIENTED_EDGE ( 'NONE', *, *, #21897, .F. ) ;
#28418=ORIENTED_EDGE ( 'NONE', *, *, #3255, .F. ) ;
#28460=VERTEX_POINT ( 'NONE', #22369 ) ;
#28477=ORIENTED_EDGE ( 'NONE', *, *, #728, .T. ) ;
#28482=VECTOR ( 'NONE', #8756, 1000.000000000000000 ) ;
#28495=DIRECTION ( 'NONE',  ( 1.000000000000000000, -1.880165489482579047E-16, 0.000000000000000000 ) ) ;
#28539=VECTOR ( 'NONE', #16208, 1000.000000000000000 ) ;
#28589=AXIS2_PLACEMENT_3D ( 'NONE', #1256, #7293, #17905 ) ;
#28594=ORIENTED_EDGE ( 'NONE', *, *, #8298, .T. ) ;
#28596=ORIENTED_EDGE ( 'NONE', *, *, #4927, .T. ) ;
#28607=DIRECTION ( 'NONE',  ( -1.880165489482579047E-16, -1.000000000000000000, -0.000000000000000000 ) ) ;
#28627=EDGE_CURVE ( 'NONE', #42219, #5125, #26129, .T. ) ;
#28676=ADVANCED_FACE ( 'NONE', ( #22831 ), #19828, .T. ) ;
#28683=AXIS2_PLACEMENT_3D ( 'NONE', #38168, #45319, #34690 ) ;
#28685=CYLINDRICAL_SURFACE ( 'NONE', #37503, 2.749999999999863665 ) ;
#28689=CARTESIAN_POINT ( 'NONE',  ( 701.1634899080286232, 259.9999999999999432, -197.2499999999991758 ) ) ;
#28705=ORIENTED_EDGE ( 'NONE', *, *, #16570, .T. ) ;
#28732=CARTESIAN_POINT ( 'NONE',  ( 959.5497976682736407, 239.9999999999998863, -209.9999999999999716 ) ) ;
#28739=CARTESIAN_POINT ( 'NONE',  ( 181.1634899080285948, 230.0000000000000000, -197.2499999999955662 ) ) ;
#28776=DIRECTION ( 'NONE',  ( 0.000000000000000000, 0.000000000000000000, 1.000000000000000000 ) ) ;
#28788=DIRECTION ( 'NONE',  ( -0.000000000000000000, 1.000000000000000000, -0.000000000000000000 ) ) ;
#28941=ORIENTED_EDGE ( 'NONE', *, *, #38237, .T. ) ;
#28947=DIRECTION ( 'NONE',  ( -1.880165489482579047E-16, -1.000000000000000000, -0.000000000000000000 ) ) ;
#28984=DIRECTION ( 'NONE',  ( -1.000000000000000000, 0.000000000000000000, 0.000000000000000000 ) ) ;
#28999=CARTESIAN_POINT ( 'NONE',  ( -911.9749999999993406, 219.9999999999998863, 350.0000000000000000 ) ) ;
#29017=CARTESIAN_POINT ( 'NONE',  ( -598.8365100919716042, 240.0000000000001705, -202.7499999999898250 ) ) ;
#29040=VECTOR ( 'NONE', #29786, 1000.000000000000000 ) ;
#29046=ORIENTED_EDGE ( 'NONE', *, *, #37087, .F. ) ;
#29059=FACE_BOUND ( 'NONE', #11630, .T. ) ;
#29080=CARTESIAN_POINT ( 'NONE',  ( -928.0249999999991815, 219.9999999999998863, 339.9999999999999432 ) ) ;
#29095=EDGE_LOOP ( 'NONE', ( #24467, #13258, #34655, #33624 ) ) ;
#29103=ORIENTED_EDGE ( 'NONE', *, *, #36433, .T. ) ;
#29134=AXIS2_PLACEMENT_3D ( 'NONE', #33111, #1448, #15549 ) ;
#29136=DIRECTION ( 'NONE',  ( 1.880165489482579047E-16, 1.000000000000000000, -0.000000000000000000 ) ) ;
#29140=DIRECTION ( 'NONE',  ( -0.000000000000000000, 1.000000000000000000, -0.000000000000000000 ) ) ;
#29147=CIRCLE ( 'NONE', #32071, 2.749999999999919176 ) ;
#29156=CARTESIAN_POINT ( 'NONE',  ( 919.9999999999993179, 154.9999999999998863, 339.9999999999999432 ) ) ;
#29161=VECTOR ( 'NONE', #29140, 1000.000000000000000 ) ;
#29163=ORIENTED_EDGE ( 'NONE', *, *, #40496, .F. ) ;
#29173=DIRECTION ( 'NONE',  ( 0.000000000000000000, 0.000000000000000000, 1.000000000000000000 ) ) ;
#29174=CARTESIAN_POINT ( 'NONE',  ( -468.8365100919714337, 260.0000000000001705, -197.2499999999910187 ) ) ;
#29182=DIRECTION ( 'NONE',  ( 1.000000000000000000, 0.000000000000000000, 0.000000000000000000 ) ) ;
#29190=DIRECTION ( 'NONE',  ( 1.880165489482579047E-16, 1.000000000000000000, -0.000000000000000000 ) ) ;
#29192=DIRECTION ( 'NONE',  ( 0.000000000000000000, 0.000000000000000000, 1.000000000000000000 ) ) ;
#29218=ADVANCED_FACE ( 'NONE', ( #43172 ), #8524, .F. ) ;
#29245=DIRECTION ( 'NONE',  ( 1.880165489482579047E-16, 1.000000000000000000, 0.000000000000000000 ) ) ;
#29263=DIRECTION ( 'NONE',  ( 1.000000000000000000, 0.000000000000000000, 0.000000000000000000 ) ) ;
#29264=DIRECTION ( 'NONE',  ( -0.000000000000000000, 1.000000000000000000, -0.000000000000000000 ) ) ;
#29278=ORIENTED_EDGE ( 'NONE', *, *, #10363, .F. ) ;
#29289=ORIENTED_EDGE ( 'NONE', *, *, #31416, .T. ) ;
#29301=DIRECTION ( 'NONE',  ( -1.880165489482579047E-16, -1.000000000000000000, 0.000000000000000000 ) ) ;
#29331=AXIS2_PLACEMENT_3D ( 'NONE', #22285, #25763, #36381 ) ;
#29456=ORIENTED_EDGE ( 'NONE', *, *, #19291, .F. ) ;
#29461=DIRECTION ( 'NONE',  ( -1.880165489482579047E-16, -1.000000000000000000, 0.000000000000000000 ) ) ;
#29466=CARTESIAN_POINT ( 'NONE',  ( -78.83651009197140525, 230.0000000000000568, -199.9999999999936051 ) ) ;
#29471=DIRECTION ( 'NONE',  ( -1.880165489482579047E-16, -1.000000000000000000, -0.000000000000000000 ) ) ;
#29492=FACE_OUTER_BOUND ( 'NONE', #24074, .T. ) ;
#29498=ADVANCED_FACE ( 'NONE', ( #23033 ), #37128, .F. ) ;
#29501=ORIENTED_EDGE ( 'NONE', *, *, #21886, .T. ) ;
#29518=DIRECTION ( 'NONE',  ( -0.000000000000000000, -0.000000000000000000, -1.000000000000000000 ) ) ;
#29525=ORIENTED_EDGE ( 'NONE', *, *, #955, .F. ) ;
#29552=EDGE_CURVE ( 'NONE', #24407, #7346, #23493, .T. ) ;
#29620=FACE_BOUND ( 'NONE', #14652, .T. ) ;
#29637=FACE_OUTER_BOUND ( 'NONE', #33864, .T. ) ;
#29692=CARTESIAN_POINT ( 'NONE',  ( -959.5497976682736407, 120.6654763175833693, -2132.806278688367456 ) ) ;
#29727=CARTESIAN_POINT ( 'NONE',  ( 831.1634899080286232, 229.9999999999998863, -199.9999999999999432 ) ) ;
#29751=EDGE_CURVE ( 'NONE', #16603, #27605, #42389, .T. ) ;
#29769=ADVANCED_FACE ( 'NONE', ( #24631, #9650, #10331, #6177, #41522 ), #38065, .F. ) ;
#29778=CIRCLE ( 'NONE', #9868, 2.749999999999919176 ) ;
#29786=DIRECTION ( 'NONE',  ( 1.000000000000000000, -1.880165489482579047E-16, 0.000000000000000000 ) ) ;
#29789=EDGE_LOOP ( 'NONE', ( #23495, #16815, #20716, #33591 ) ) ;
#29834=ORIENTED_EDGE ( 'NONE', *, *, #17111, .T. ) ;
#29837=ORIENTED_EDGE ( 'NONE', *, *, #7143, .F. ) ;
#29845=LINE ( 'NONE', #26149, #6965 ) ;
#29852=DIRECTION ( 'NONE',  ( 1.000000000000000000, 0.000000000000000000, 0.000000000000000000 ) ) ;
#29873=VECTOR ( 'NONE', #44175, 1000.000000000000000 ) ;
#29889=CIRCLE ( 'NONE', #35803, 8.024999999999948841 ) ;
#29894=CIRCLE ( 'NONE', #18840, 8.024999999999948841 ) ;
#29895=ORIENTED_EDGE ( 'NONE', *, *, #8337, .F. ) ;
#29921=AXIS2_PLACEMENT_3D ( 'NONE', #14235, #28304, #34784 ) ;
#29926=AXIS2_PLACEMENT_3D ( 'NONE', #25506, #17680, #35903 ) ;
#29931=EDGE_LOOP ( 'NONE', ( #24939, #4615 ) ) ;
#29953=CARTESIAN_POINT ( 'NONE',  ( -521.6730038022808458, 200.0000000000001421, -122.7905160835438068 ) ) ;
#29965=CARTESIAN_POINT ( 'NONE',  ( -728.8365100919714905, 240.0000000000001990, -202.7499999999889440 ) ) ;
#29992=VECTOR ( 'NONE', #40137, 1000.000000000000000 ) ;
#30011=DIRECTION ( 'NONE',  ( 1.000000000000000000, 0.000000000000000000, 0.000000000000000000 ) ) ;
#30034=EDGE_CURVE ( 'NONE', #12718, #44771, #29147, .T. ) ;
#30063=EDGE_LOOP ( 'NONE', ( #32664, #13475 ) ) ;
#30067=VERTEX_POINT ( 'NONE', #18418 ) ;
#30092=DIRECTION ( 'NONE',  ( -1.880165489482579047E-16, -1.000000000000000000, 0.000000000000000000 ) ) ;
#30107=EDGE_LOOP ( 'NONE', ( #25951, #4724, #35178, #13878, #29046, #15253, #40644, #45526 ) ) ;
#30152=VECTOR ( 'NONE', #4094, 1000.000000000000000 ) ;
#30153=CARTESIAN_POINT ( 'NONE',  ( 571.1634899080285095, 239.9999999999999716, -199.9999999999981526 ) ) ;
#30157=ORIENTED_EDGE ( 'NONE', *, *, #16185, .T. ) ;
#30211=LINE ( 'NONE', #23498, #44706 ) ;
#30232=ORIENTED_EDGE ( 'NONE', *, *, #34849, .F. ) ;
#30250=CARTESIAN_POINT ( 'NONE',  ( 959.5497976682736407, 239.9999999999998863, 350.0000000000000000 ) ) ;
#30270=ORIENTED_EDGE ( 'NONE', *, *, #39742, .T. ) ;
#30273=ORIENTED_EDGE ( 'NONE', *, *, #1182, .F. ) ;
#30288=CARTESIAN_POINT ( 'NONE',  ( -468.8365100919714337, 230.0000000000001421, -197.2499999999910187 ) ) ;
#30289=EDGE_CURVE ( 'NONE', #9329, #44845, #23972, .T. ) ;
#30315=ORIENTED_EDGE ( 'NONE', *, *, #37138, .F. ) ;
#30331=ORIENTED_EDGE ( 'NONE', *, *, #16185, .F. ) ;
#30344=CARTESIAN_POINT ( 'NONE',  ( 701.1634899080286232, 229.9999999999999147, -197.2499999999991758 ) ) ;
#30363=DIRECTION ( 'NONE',  ( -0.000000000000000000, -0.000000000000000000, 1.000000000000000000 ) ) ;
#30375=CARTESIAN_POINT ( 'NONE',  ( -454.7528517110260964, 200.0000000000001137, -122.7905160835438068 ) ) ;
#30383=AXIS2_PLACEMENT_3D ( 'NONE', #25545, #18620, #25306 ) ;
#30386=EDGE_LOOP ( 'NONE', ( #5496, #30315 ) ) ;
#30400=LINE ( 'NONE', #29953, #20314 ) ;
#30440=CARTESIAN_POINT ( 'NONE',  ( -468.8365100919714337, 240.0000000000001705, -199.9999999999908766 ) ) ;
#30479=LINE ( 'NONE', #6225, #21322 ) ;
#30499=AXIS2_PLACEMENT_3D ( 'NONE', #14293, #39020, #14070 ) ;
#30517=DIRECTION ( 'NONE',  ( -1.880165489482579047E-16, -1.000000000000000000, -0.000000000000000000 ) ) ;
#30518=VERTEX_POINT ( 'NONE', #44469 ) ;
#30520=EDGE_CURVE ( 'NONE', #27605, #16603, #4812, .T. ) ;
#30543=LINE ( 'NONE', #27995, #1149 ) ;
#30571=EDGE_CURVE ( 'NONE', #14331, #42109, #9373, .T. ) ;
#30574=DIRECTION ( 'NONE',  ( -1.000000000000000000, 0.000000000000000000, 0.000000000000000000 ) ) ;
#30595=DIRECTION ( 'NONE',  ( -1.000000000000000000, 1.880165489482579047E-16, 0.000000000000000000 ) ) ;
#30616=EDGE_CURVE ( 'NONE', #20005, #33196, #31378, .T. ) ;
#30627=CIRCLE ( 'NONE', #25486, 2.749999999999808153 ) ;
#30651=CARTESIAN_POINT ( 'NONE',  ( -468.8365100919714337, 240.0000000000001705, -197.2499999999910187 ) ) ;
#30664=CARTESIAN_POINT ( 'NONE',  ( -598.8365100919716042, 260.0000000000001705, -199.9999999999899671 ) ) ;
#30666=ORIENTED_EDGE ( 'NONE', *, *, #43810, .T. ) ;
#30681=AXIS2_PLACEMENT_3D ( 'NONE', #43025, #42584, #38902 ) ;
#30705=LINE ( 'NONE', #10142, #12697 ) ;
#30746=PRODUCT_CONTEXT ( 'NONE', #43487, 'mechanical' ) ;
#30812=ORIENTED_EDGE ( 'NONE', *, *, #42786, .T. ) ;
#30879=CARTESIAN_POINT ( 'NONE',  ( 928.0249999999991815, 154.9999999999998863, 339.9999999999999432 ) ) ;
#30880=CYLINDRICAL_SURFACE ( 'NONE', #7573, 2.749999999999863665 ) ;
#30891=FACE_OUTER_BOUND ( 'NONE', #3069, .T. ) ;
#30947=LINE ( 'NONE', #41566, #40927 ) ;
#31069=CARTESIAN_POINT ( 'NONE',  ( -338.8365100919713200, 260.0000000000001137, -199.9999999999917861 ) ) ;
#31096=DIRECTION ( 'NONE',  ( -0.000000000000000000, 1.000000000000000000, -0.000000000000000000 ) ) ;
#31129=EDGE_LOOP ( 'NONE', ( #20576, #13357, #35493, #45286 ) ) ;
#31158=ADVANCED_FACE ( 'NONE', ( #10975 ), #7973, .F. ) ;
#31178=EDGE_CURVE ( 'NONE', #27330, #5332, #29889, .T. ) ;
#31182=EDGE_LOOP ( 'NONE', ( #20109, #28705, #43363, #12500 ) ) ;
#31278=CARTESIAN_POINT ( 'NONE',  ( -521.6730038022808458, 200.0000000000001421, -122.7905160835438068 ) ) ;
#31350=AXIS2_PLACEMENT_3D ( 'NONE', #37541, #19988, #34064 ) ;
#31358=VECTOR ( 'NONE', #23819, 1000.000000000000000 ) ;
#31361=AXIS2_PLACEMENT_3D ( 'NONE', #4357, #28607, #43148 ) ;
#31365=ORIENTED_EDGE ( 'NONE', *, *, #41330, .F. ) ;
#31378=CIRCLE ( 'NONE', #8513, 2.749999999999919176 ) ;
#31393=EDGE_CURVE ( 'NONE', #15014, #13142, #39553, .T. ) ;
#31396=DIRECTION ( 'NONE',  ( -0.000000000000000000, 1.000000000000000000, -0.000000000000000000 ) ) ;
#31416=EDGE_CURVE ( 'NONE', #41897, #21010, #4841, .T. ) ;
#31438=ORIENTED_EDGE ( 'NONE', *, *, #17957, .F. ) ;
#31494=CARTESIAN_POINT ( 'NONE',  ( -521.6730038022808458, 230.0000000000002274, 339.9999999999999432 ) ) ;
#31498=DIRECTION ( 'NONE',  ( -1.880165489482579047E-16, -1.000000000000000000, -0.000000000000000000 ) ) ;
#31507=DIRECTION ( 'NONE',  ( -0.000000000000000000, 1.000000000000000000, -0.000000000000000000 ) ) ;
#31528=ADVANCED_BREP_SHAPE_REPRESENTATION ( '', ( #32965, #26858 ), #32022 ) ;
#31564=CYLINDRICAL_SURFACE ( 'NONE', #1141, 2.749999999999863665 ) ;
#31566=CARTESIAN_POINT ( 'NONE',  ( 959.5497976682736407, 229.9999999999998579, -122.7905160835436362 ) ) ;
#31577=DIRECTION ( 'NONE',  ( 0.000000000000000000, 0.000000000000000000, 1.000000000000000000 ) ) ;
#31652=ORIENTED_EDGE ( 'NONE', *, *, #2160, .T. ) ;
#31657=CARTESIAN_POINT ( 'NONE',  ( 831.1634899080286232, 239.9999999999999147, -199.9999999999999432 ) ) ;
#31673=PLANE ( 'NONE',  #28683 ) ;
#31747=CYLINDRICAL_SURFACE ( 'NONE', #35205, 2.749999999999863665 ) ;
#31779=DIRECTION ( 'NONE',  ( -1.880165489482579047E-16, -1.000000000000000000, -0.000000000000000000 ) ) ;
#31801=AXIS2_PLACEMENT_3D ( 'NONE', #33990, #33775, #29852 ) ;
#31875=CARTESIAN_POINT ( 'NONE',  ( 181.1634899080285948, 260.0000000000000000, -199.9999999999953957 ) ) ;
#31882=VECTOR ( 'NONE', #19339, 1000.000000000000000 ) ;
#31928=EDGE_LOOP ( 'NONE', ( #11622, #5802 ) ) ;
#31932=FACE_OUTER_BOUND ( 'NONE', #7007, .T. ) ;
#31933=ADVANCED_FACE ( 'NONE', ( #41187 ), #2362, .F. ) ;
#31937=DIRECTION ( 'NONE',  ( -0.000000000000000000, -0.000000000000000000, 1.000000000000000000 ) ) ;
#31938=ORIENTED_EDGE ( 'NONE', *, *, #32500, .F. ) ;
#32022=( GEOMETRIC_REPRESENTATION_CONTEXT ( 3 ) GLOBAL_UNCERTAINTY_ASSIGNED_CONTEXT ( ( #1468 ) ) GLOBAL_UNIT_ASSIGNED_CONTEXT ( ( #40729, #22722, #33804 ) ) REPRESENTATION_CONTEXT ( 'NONE', 'WORKASPACE' ) );
#32023=VECTOR ( 'NONE', #21796, 1000.000000000000000 ) ;
#32059=DIRECTION ( 'NONE',  ( -0.000000000000000000, -0.000000000000000000, 1.000000000000000000 ) ) ;
#32071=AXIS2_PLACEMENT_3D ( 'NONE', #36184, #15406, #42428 ) ;
#32074=VECTOR ( 'NONE', #23439, 1000.000000000000000 ) ;
#32139=AXIS2_PLACEMENT_3D ( 'NONE', #9541, #34702, #20607 ) ;
#32183=VECTOR ( 'NONE', #18718, 1000.000000000000000 ) ;
#32247=DIRECTION ( 'NONE',  ( -0.000000000000000000, 1.000000000000000000, -0.000000000000000000 ) ) ;
#32258=DIRECTION ( 'NONE',  ( -0.000000000000000000, 1.000000000000000000, -0.000000000000000000 ) ) ;
#32272=DIRECTION ( 'NONE',  ( -1.880165489482579047E-16, -1.000000000000000000, -0.000000000000000000 ) ) ;
#32312=ORIENTED_EDGE ( 'NONE', *, *, #728, .F. ) ;
#32332=EDGE_CURVE ( 'NONE', #5125, #42219, #11549, .T. ) ;
#32364=EDGE_CURVE ( 'NONE', #43290, #7811, #15004, .T. ) ;
#32370=LINE ( 'NONE', #8122, #38619 ) ;
#32399=ORIENTED_EDGE ( 'NONE', *, *, #10302, .T. ) ;
#32406=VERTEX_POINT ( 'NONE', #5492 ) ;
#32428=FACE_OUTER_BOUND ( 'NONE', #39244, .T. ) ;
#32430=CARTESIAN_POINT ( 'NONE',  ( 959.5497976682736407, 120.6654763175833693, 350.0000000000000000 ) ) ;
#32463=ORIENTED_EDGE ( 'NONE', *, *, #34849, .T. ) ;
#32500=EDGE_CURVE ( 'NONE', #20516, #2099, #30211, .T. ) ;
#32532=DIRECTION ( 'NONE',  ( -0.000000000000000000, 1.000000000000000000, -0.000000000000000000 ) ) ;
#32578=VERTEX_POINT ( 'NONE', #12657 ) ;
#32606=CARTESIAN_POINT ( 'NONE',  ( 311.1634899080286232, 260.0000000000000000, -197.2499999999964473 ) ) ;
#32624=EDGE_CURVE ( 'NONE', #42970, #14331, #9656, .T. ) ;
#32663=FACE_BOUND ( 'NONE', #30386, .T. ) ;
#32664=ORIENTED_EDGE ( 'NONE', *, *, #30520, .F. ) ;
#32683=VERTEX_POINT ( 'NONE', #6865 ) ;
#32697=CARTESIAN_POINT ( 'NONE',  ( -598.8365100919716042, 240.0000000000001705, -197.2499999999901092 ) ) ;
#32752=CARTESIAN_POINT ( 'NONE',  ( -338.8365100919713200, 230.0000000000001137, -202.7499999999916724 ) ) ;
#32773=DIRECTION ( 'NONE',  ( 0.000000000000000000, 0.000000000000000000, 1.000000000000000000 ) ) ;
#32784=CARTESIAN_POINT ( 'NONE',  ( -468.8365100919714337, 240.0000000000001705, -199.9999999999908766 ) ) ;
#32808=AXIS2_PLACEMENT_3D ( 'NONE', #8852, #30092, #8401 ) ;
#32947=CYLINDRICAL_SURFACE ( 'NONE', #5433, 2.749999999999863665 ) ;
#32949=ADVANCED_FACE ( 'NONE', ( #29492 ), #32969, .F. ) ;
#32965=MANIFOLD_SOLID_BREP ( 'Cut-Extrude9', #10692 ) ;
#32969=CYLINDRICAL_SURFACE ( 'NONE', #26780, 2.749999999999863665 ) ;
#32972=ORIENTED_EDGE ( 'NONE', *, *, #32364, .T. ) ;
#33047=VECTOR ( 'NONE', #25899, 1000.000000000000000 ) ;
#33111=CARTESIAN_POINT ( 'NONE',  ( -728.8365100919714905, 230.0000000000001705, -199.9999999999890861 ) ) ;
#33139=CARTESIAN_POINT ( 'NONE',  ( 571.1634899080285095, 229.9999999999999432, -199.9999999999981526 ) ) ;
#33150=EDGE_CURVE ( 'NONE', #15014, #1382, #23447, .T. ) ;
#33175=CARTESIAN_POINT ( 'NONE',  ( 454.7528517110262101, 229.9999999999999432, -122.7905160835442615 ) ) ;
#33182=CARTESIAN_POINT ( 'NONE',  ( 571.1634899080285095, 229.9999999999999432, -199.9999999999981526 ) ) ;
#33196=VERTEX_POINT ( 'NONE', #19770 ) ;
#33351=ORIENTED_EDGE ( 'NONE', *, *, #25533, .F. ) ;
#33371=VECTOR ( 'NONE', #12866, 1000.000000000000000 ) ;
#33380=DIRECTION ( 'NONE',  ( -1.880165489482579047E-16, -1.000000000000000000, -0.000000000000000000 ) ) ;
#33385=DIRECTION ( 'NONE',  ( -0.000000000000000000, 1.000000000000000000, -0.000000000000000000 ) ) ;
#33397=VERTEX_POINT ( 'NONE', #5906 ) ;
#33448=DIRECTION ( 'NONE',  ( 1.000000000000000000, -1.880165489482579047E-16, 0.000000000000000000 ) ) ;
#33468=EDGE_LOOP ( 'NONE', ( #25708, #24376, #38640, #12012 ) ) ;
#33487=DIRECTION ( 'NONE',  ( -1.880165489482579047E-16, -1.000000000000000000, -0.000000000000000000 ) ) ;
#33536=EDGE_LOOP ( 'NONE', ( #5626, #6437, #28477, #42777 ) ) ;
#33570=VERTEX_POINT ( 'NONE', #41475 ) ;
#33574=CARTESIAN_POINT ( 'NONE',  ( -454.7528517110260964, 200.0000000000001137, 339.9999999999999432 ) ) ;
#33587=VECTOR ( 'NONE', #44878, 1000.000000000000000 ) ;
#33591=ORIENTED_EDGE ( 'NONE', *, *, #43788, .F. ) ;
#33603=CIRCLE ( 'NONE', #13702, 2.749999999999919176 ) ;
#33620=CARTESIAN_POINT ( 'NONE',  ( 311.1634899080286232, 260.0000000000000000, -202.7499999999961915 ) ) ;
#33624=ORIENTED_EDGE ( 'NONE', *, *, #5239, .T. ) ;
#33658=DIRECTION ( 'NONE',  ( 0.000000000000000000, 0.000000000000000000, 1.000000000000000000 ) ) ;
#33692=DIRECTION ( 'NONE',  ( -1.000000000000000000, 4.147566128926370535E-16, 0.000000000000000000 ) ) ;
#33702=VERTEX_POINT ( 'NONE', #2675 ) ;
#33708=ADVANCED_FACE ( 'NONE', ( #38461 ), #31747, .F. ) ;
#33712=EDGE_CURVE ( 'NONE', #1685, #10345, #13091, .T. ) ;
#33769=EDGE_CURVE ( 'NONE', #5289, #20839, #8678, .T. ) ;
#33770=DIRECTION ( 'NONE',  ( 1.000000000000000000, 0.000000000000000000, 0.000000000000000000 ) ) ;
#33775=DIRECTION ( 'NONE',  ( -1.880165489482579047E-16, -1.000000000000000000, -0.000000000000000000 ) ) ;
#33779=DIRECTION ( 'NONE',  ( -1.880165489482579047E-16, -1.000000000000000000, -0.000000000000000000 ) ) ;
#33782=AXIS2_PLACEMENT_3D ( 'NONE', #39054, #35799, #3710 ) ;
#33804=( NAMED_UNIT ( * ) SI_UNIT ( $, .STERADIAN. ) SOLID_ANGLE_UNIT ( ) );
#33817=DIRECTION ( 'NONE',  ( 0.000000000000000000, 0.000000000000000000, 1.000000000000000000 ) ) ;
#33848=DIRECTION ( 'NONE',  ( 0.000000000000000000, 0.000000000000000000, -1.000000000000000000 ) ) ;
#33864=EDGE_LOOP ( 'NONE', ( #10837, #43029, #24220, #12248, #18761, #26755, #29163, #40118, #16146, #39688, #13984, #31938 ) ) ;
#33904=DIRECTION ( 'NONE',  ( 1.880165489482579047E-16, 1.000000000000000000, 0.000000000000000000 ) ) ;
#33913=ORIENTED_EDGE ( 'NONE', *, *, #9206, .F. ) ;
#33927=CARTESIAN_POINT ( 'NONE',  ( 959.5497976682736407, 229.9999999999998579, 339.9999999999998863 ) ) ;
#33929=CARTESIAN_POINT ( 'NONE',  ( 959.5497976682736407, 229.9999999999998579, 339.9999999999998863 ) ) ;
#33957=VERTEX_POINT ( 'NONE', #43511 ) ;
#33975=ORIENTED_EDGE ( 'NONE', *, *, #18712, .F. ) ;
#33989=EDGE_CURVE ( 'NONE', #17477, #791, #18995, .T. ) ;
#33990=CARTESIAN_POINT ( 'NONE',  ( 311.1634899080286232, 229.9999999999999716, -199.9999999999963336 ) ) ;
#33993=CARTESIAN_POINT ( 'NONE',  ( 51.16348990802859475, 240.0000000000000568, -199.9999999999945146 ) ) ;
#34012=EDGE_CURVE ( 'NONE', #33397, #3427, #4974, .T. ) ;
#34026=ORIENTED_EDGE ( 'NONE', *, *, #43817, .T. ) ;
#34033=PLANE ( 'NONE',  #16171 ) ;
#34036=DIRECTION ( 'NONE',  ( -0.000000000000000000, -0.000000000000000000, -1.000000000000000000 ) ) ;
#34037=DIRECTION ( 'NONE',  ( 0.000000000000000000, 0.000000000000000000, 1.000000000000000000 ) ) ;
#34064=DIRECTION ( 'NONE',  ( 1.000000000000000000, 0.000000000000000000, 0.000000000000000000 ) ) ;
#34096=CARTESIAN_POINT ( 'NONE',  ( -949.5497976682736407, 230.0000000000002274, 339.9999999999999432 ) ) ;
#34106=DIRECTION ( 'NONE',  ( 1.000000000000000000, 0.000000000000000000, 0.000000000000000000 ) ) ;
#34123=ORIENTED_EDGE ( 'NONE', *, *, #42732, .T. ) ;
#34128=ORIENTED_EDGE ( 'NONE', *, *, #25747, .F. ) ;
#34137=EDGE_LOOP ( 'NONE', ( #26187, #874, #27906, #36600 ) ) ;
#34139=CARTESIAN_POINT ( 'NONE',  ( 959.5497976682736407, 239.9999999999998863, -209.9999999999999716 ) ) ;
#34173=VERTEX_POINT ( 'NONE', #10983 ) ;
#34211=DIRECTION ( 'NONE',  ( -0.000000000000000000, -0.000000000000000000, -1.000000000000000000 ) ) ;
#34226=CARTESIAN_POINT ( 'NONE',  ( -454.7528517110262101, 230.0000000000001421, -2132.806278688367456 ) ) ;
#34241=DIRECTION ( 'NONE',  ( 0.000000000000000000, 0.000000000000000000, 1.000000000000000000 ) ) ;
#34262=CIRCLE ( 'NONE', #23208, 2.749999999999863665 ) ;
#34278=CARTESIAN_POINT ( 'NONE',  ( -454.7528517110261532, 8.550106180308601742E-14, 339.9999999999999432 ) ) ;
#34391=EDGE_LOOP ( 'NONE', ( #17267, #39509, #18448, #22214, #44095, #33975 ) ) ;
#34406=LINE ( 'NONE', #2775, #40215 ) ;
#34429=DIRECTION ( 'NONE',  ( 1.000000000000000000, -1.880165489482579047E-16, 0.000000000000000000 ) ) ;
#34444=VECTOR ( 'NONE', #39345, 1000.000000000000000 ) ;
#34446=CARTESIAN_POINT ( 'NONE',  ( -208.8365100919714052, 230.0000000000000853, -197.2499999999928377 ) ) ;
#34478=CARTESIAN_POINT ( 'NONE',  ( -911.9749999999993406, 219.9999999999998863, -360.0000000000000000 ) ) ;
#34524=FACE_OUTER_BOUND ( 'NONE', #4617, .T. ) ;
#34530=CARTESIAN_POINT ( 'NONE',  ( -959.5497976682736407, 240.0000000000002274, 350.0000000000000000 ) ) ;
#34553=ORIENTED_EDGE ( 'NONE', *, *, #33712, .F. ) ;
#34573=CARTESIAN_POINT ( 'NONE',  ( 311.1634899080286232, 260.0000000000000000, -199.9999999999963336 ) ) ;
#34593=DIRECTION ( 'NONE',  ( -1.000000000000000000, 0.000000000000000000, 0.000000000000000000 ) ) ;
#34607=EDGE_LOOP ( 'NONE', ( #2710, #43820 ) ) ;
#34625=CARTESIAN_POINT ( 'NONE',  ( -919.9999999999993179, 219.9999999999998863, -360.0000000000000000 ) ) ;
#34655=ORIENTED_EDGE ( 'NONE', *, *, #39901, .F. ) ;
#34665=ADVANCED_FACE ( 'NONE', ( #3301 ), #38190, .F. ) ;
#34678=ORIENTED_EDGE ( 'NONE', *, *, #15877, .T. ) ;
#34690=DIRECTION ( 'NONE',  ( 0.000000000000000000, 0.000000000000000000, -1.000000000000000000 ) ) ;
#34702=DIRECTION ( 'NONE',  ( -0.000000000000000000, 1.000000000000000000, -0.000000000000000000 ) ) ;
#34718=EDGE_LOOP ( 'NONE', ( #15617, #21967 ) ) ;
#34747=CARTESIAN_POINT ( 'NONE',  ( -468.8365100919714337, 230.0000000000001421, -202.7499999999907345 ) ) ;
#34784=DIRECTION ( 'NONE',  ( 1.000000000000000000, 0.000000000000000000, 0.000000000000000000 ) ) ;
#34820=EDGE_CURVE ( 'NONE', #30067, #39336, #45583, .T. ) ;
#34841=EDGE_LOOP ( 'NONE', ( #27334, #8424, #36976, #43072 ) ) ;
#34849=EDGE_CURVE ( 'NONE', #15138, #12788, #23416, .T. ) ;
#34897=LINE ( 'NONE', #17356, #23949 ) ;
#34919=CIRCLE ( 'NONE', #15020, 2.749999999999835687 ) ;
#34925=AXIS2_PLACEMENT_3D ( 'NONE', #31657, #39532, #21964 ) ;
#34926=LINE ( 'NONE', #34226, #24712 ) ;
#34933=EDGE_LOOP ( 'NONE', ( #37714, #12654, #31365, #25821 ) ) ;
#34955=ORIENTED_EDGE ( 'NONE', *, *, #8497, .F. ) ;
#34968=CARTESIAN_POINT ( 'NONE',  ( 949.5497976682736407, 120.6654763175833693, -209.9999999999999716 ) ) ;
#34985=AXIS2_PLACEMENT_3D ( 'NONE', #19256, #37262, #2616 ) ;
#34999=ORIENTED_EDGE ( 'NONE', *, *, #39673, .F. ) ;
#35022=EDGE_CURVE ( 'NONE', #27330, #9635, #24769, .T. ) ;
#35133=VECTOR ( 'NONE', #26759, 1000.000000000000000 ) ;
#35178=ORIENTED_EDGE ( 'NONE', *, *, #41944, .T. ) ;
#35184=CARTESIAN_POINT ( 'NONE',  ( 181.1634899080285948, 230.0000000000000000, -202.7499999999952536 ) ) ;
#35205=AXIS2_PLACEMENT_3D ( 'NONE', #31069, #24134, #44947 ) ;
#35251=CARTESIAN_POINT ( 'NONE',  ( 181.1634899080285948, 240.0000000000000284, -199.9999999999953957 ) ) ;
#35263=CARTESIAN_POINT ( 'NONE',  ( -78.83651009197140525, 260.0000000000000568, -199.9999999999936051 ) ) ;
#35317=FACE_BOUND ( 'NONE', #20393, .T. ) ;
#35323=EDGE_CURVE ( 'NONE', #44845, #44771, #36760, .T. ) ;
#35326=AXIS2_PLACEMENT_3D ( 'NONE', #6916, #42033, #21462 ) ;
#35334=ORIENTED_EDGE ( 'NONE', *, *, #41924, .T. ) ;
#35388=ORIENTED_EDGE ( 'NONE', *, *, #5139, .T. ) ;
#35455=VERTEX_POINT ( 'NONE', #24473 ) ;
#35464=CARTESIAN_POINT ( 'NONE',  ( 911.9749999999993406, 154.9999999999998863, 339.9999999999999432 ) ) ;
#35493=ORIENTED_EDGE ( 'NONE', *, *, #8337, .T. ) ;
#35525=ORIENTED_EDGE ( 'NONE', *, *, #1802, .T. ) ;
#35593=CARTESIAN_POINT ( 'NONE',  ( 9.202092513630239068E-14, 199.9999999999999147, 0.000000000000000000 ) ) ;
#35633=CARTESIAN_POINT ( 'NONE',  ( -78.83651009197140525, 240.0000000000000853, -199.9999999999936051 ) ) ;
#35661=ADVANCED_FACE ( 'NONE', ( #9497 ), #16658, .F. ) ;
#35668=CARTESIAN_POINT ( 'NONE',  ( -468.8365100919714337, 230.0000000000001421, -199.9999999999908766 ) ) ;
#35690=ORIENTED_EDGE ( 'NONE', *, *, #37965, .F. ) ;
#35715=CARTESIAN_POINT ( 'NONE',  ( 8.295132257852724189E-14, 199.9999999999999147, 350.0000000000000000 ) ) ;
#35717=CIRCLE ( 'NONE', #8425, 2.749999999999835687 ) ;
#35740=ORIENTED_EDGE ( 'NONE', *, *, #24640, .F. ) ;
#35761=CARTESIAN_POINT ( 'NONE',  ( 959.5497976682736407, 120.6654763175833693, 350.0000000000000000 ) ) ;
#35799=DIRECTION ( 'NONE',  ( 0.000000000000000000, 0.000000000000000000, 1.000000000000000000 ) ) ;
#35803=AXIS2_PLACEMENT_3D ( 'NONE', #796, #14201, #38935 ) ;
#35860=ORIENTED_EDGE ( 'NONE', *, *, #6919, .F. ) ;
#35903=DIRECTION ( 'NONE',  ( 1.000000000000000000, 0.000000000000000000, 0.000000000000000000 ) ) ;
#35921=ORIENTED_EDGE ( 'NONE', *, *, #23535, .T. ) ;
#35926=AXIS2_PLACEMENT_3D ( 'NONE', #43155, #25605, #12192 ) ;
#35941=CARTESIAN_POINT ( 'NONE',  ( 441.1634899080286232, 259.9999999999999432, -202.7499999999971010 ) ) ;
#35945=EDGE_CURVE ( 'NONE', #282, #928, #37473, .T. ) ;
#35955=DIRECTION ( 'NONE',  ( 0.000000000000000000, 0.000000000000000000, 1.000000000000000000 ) ) ;
#36050=CARTESIAN_POINT ( 'NONE',  ( -949.5497976682736407, 230.0000000000002274, -2132.806278688367456 ) ) ;
#36087=CARTESIAN_POINT ( 'NONE',  ( 51.16348990802859475, 260.0000000000000568, -202.7499999999943441 ) ) ;
#36103=DIRECTION ( 'NONE',  ( -0.000000000000000000, 1.000000000000000000, -0.000000000000000000 ) ) ;
#36110=DIRECTION ( 'NONE',  ( -1.880165489482579047E-16, -1.000000000000000000, -0.000000000000000000 ) ) ;
#36167=DIRECTION ( 'NONE',  ( -1.880165489482579047E-16, -1.000000000000000000, -0.000000000000000000 ) ) ;
#36184=CARTESIAN_POINT ( 'NONE',  ( -598.8365100919716042, 240.0000000000001705, -199.9999999999899671 ) ) ;
#36262=ADVANCED_FACE ( 'NONE', ( #30891 ), #13566, .F. ) ;
#36267=LINE ( 'NONE', #18954, #29040 ) ;
#36287=CARTESIAN_POINT ( 'NONE',  ( -468.8365100919714337, 260.0000000000001705, -199.9999999999908766 ) ) ;
#36343=FACE_BOUND ( 'NONE', #6189, .T. ) ;
#36381=DIRECTION ( 'NONE',  ( 0.000000000000000000, 0.000000000000000000, 1.000000000000000000 ) ) ;
#36412=DIRECTION ( 'NONE',  ( 0.000000000000000000, 0.000000000000000000, 1.000000000000000000 ) ) ;
#36415=EDGE_LOOP ( 'NONE', ( #25852, #11886 ) ) ;
#36423=VECTOR ( 'NONE', #28495, 1000.000000000000000 ) ;
#36433=EDGE_CURVE ( 'NONE', #11158, #44330, #28321, .T. ) ;
#36448=PLANE ( 'NONE',  #24871 ) ;
#36547=ORIENTED_EDGE ( 'NONE', *, *, #38237, .F. ) ;
#36566=AXIS2_PLACEMENT_3D ( 'NONE', #4515, #1040, #15145 ) ;
#36587=EDGE_LOOP ( 'NONE', ( #15974, #37446 ) ) ;
#36600=ORIENTED_EDGE ( 'NONE', *, *, #32332, .F. ) ;
#36664=AXIS2_PLACEMENT_3D ( 'NONE', #17932, #32247, #43322 ) ;
#36695=ORIENTED_EDGE ( 'NONE', *, *, #30520, .T. ) ;
#36696=EDGE_CURVE ( 'NONE', #22008, #12108, #21633, .T. ) ;
#36718=EDGE_LOOP ( 'NONE', ( #18548, #38760, #22940, #35740 ) ) ;
#36724=CYLINDRICAL_SURFACE ( 'NONE', #20903, 2.749999999999863665 ) ;
#36734=DIRECTION ( 'NONE',  ( 1.000000000000000000, 0.000000000000000000, 0.000000000000000000 ) ) ;
#36760=LINE ( 'NONE', #40673, #33047 ) ;
#36769=ADVANCED_FACE ( 'NONE', ( #15174 ), #25319, .F. ) ;
#36777=CARTESIAN_POINT ( 'NONE',  ( -949.5497976682736407, 240.0000000000002274, -209.9999999999999716 ) ) ;
#36780=DIRECTION ( 'NONE',  ( 1.000000000000000000, 0.000000000000000000, 0.000000000000000000 ) ) ;
#36818=SHAPE_REPRESENTATION_RELATIONSHIP ( 'NONE' , 'NONE' ,  #18903, #31528 ) ;
#36831=VERTEX_POINT ( 'NONE', #25989 ) ;
#36833=DIRECTION ( 'NONE',  ( 1.000000000000000000, 0.000000000000000000, 0.000000000000000000 ) ) ;
#36843=DIRECTION ( 'NONE',  ( 1.000000000000000000, 0.000000000000000000, 0.000000000000000000 ) ) ;
#36881=ORIENTED_EDGE ( 'NONE', *, *, #36894, .F. ) ;
#36894=EDGE_CURVE ( 'NONE', #32406, #23058, #22052, .T. ) ;
#36899=ORIENTED_EDGE ( 'NONE', *, *, #7510, .F. ) ;
#36912=EDGE_LOOP ( 'NONE', ( #5446, #13872, #16940, #13786, #36938, #10235, #35860, #30331, #38080, #26639, #18019, #11769 ) ) ;
#36927=ORIENTED_EDGE ( 'NONE', *, *, #27798, .F. ) ;
#36935=EDGE_LOOP ( 'NONE', ( #7516, #35525, #44726, #14149 ) ) ;
#36938=ORIENTED_EDGE ( 'NONE', *, *, #36696, .F. ) ;
#36976=ORIENTED_EDGE ( 'NONE', *, *, #5541, .F. ) ;
#37010=FACE_BOUND ( 'NONE', #1199, .T. ) ;
#37011=CARTESIAN_POINT ( 'NONE',  ( 959.5497976682736407, 239.9999999999998863, 350.0000000000000000 ) ) ;
#37030=LINE ( 'NONE', #5384, #40146 ) ;
#37046=CARTESIAN_POINT ( 'NONE',  ( -858.8365100919713768, 230.0000000000001990, -197.2499999999882903 ) ) ;
#37087=EDGE_CURVE ( 'NONE', #13538, #5955, #9751, .T. ) ;
#37093=ORIENTED_EDGE ( 'NONE', *, *, #42786, .F. ) ;
#37122=ORIENTED_EDGE ( 'NONE', *, *, #955, .T. ) ;
#37128=CYLINDRICAL_SURFACE ( 'NONE', #1818, 8.024999999999948841 ) ;
#37136=ORIENTED_EDGE ( 'NONE', *, *, #8252, .T. ) ;
#37138=EDGE_CURVE ( 'NONE', #38643, #12556, #13941, .T. ) ;
#37171=AXIS2_PLACEMENT_3D ( 'NONE', #990, #14178, #43263 ) ;
#37173=DIRECTION ( 'NONE',  ( 1.000000000000000000, 0.000000000000000000, 0.000000000000000000 ) ) ;
#37180=DIRECTION ( 'NONE',  ( -1.880165489482579047E-16, -1.000000000000000000, -0.000000000000000000 ) ) ;
#37219=CARTESIAN_POINT ( 'NONE',  ( 454.7528517110262101, 199.9999999999999432, -122.7905160835442615 ) ) ;
#37254=ADVANCED_FACE ( 'NONE', ( #42079 ), #31673, .F. ) ;
#37262=DIRECTION ( 'NONE',  ( -0.000000000000000000, 1.000000000000000000, -0.000000000000000000 ) ) ;
#37266=VECTOR ( 'NONE', #45666, 1000.000000000000000 ) ;
#37274=CARTESIAN_POINT ( 'NONE',  ( -928.0249999999991815, 154.9999999999998863, 350.0000000000000000 ) ) ;
#37275=FACE_OUTER_BOUND ( 'NONE', #33536, .T. ) ;
#37293=DIRECTION ( 'NONE',  ( -0.000000000000000000, 0.000000000000000000, 1.000000000000000000 ) ) ;
#37310=DIRECTION ( 'NONE',  ( -1.880165489482579047E-16, -1.000000000000000000, -0.000000000000000000 ) ) ;
#37338=LINE ( 'NONE', #12852, #10735 ) ;
#37400=ORIENTED_EDGE ( 'NONE', *, *, #27454, .T. ) ;
#37413=ADVANCED_FACE ( 'NONE', ( #22194 ), #28685, .F. ) ;
#37446=ORIENTED_EDGE ( 'NONE', *, *, #42732, .F. ) ;
#37473=CIRCLE ( 'NONE', #33782, 8.024999999999948841 ) ;
#37475=DIRECTION ( 'NONE',  ( -1.880165489482579047E-16, -1.000000000000000000, -0.000000000000000000 ) ) ;
#37503=AXIS2_PLACEMENT_3D ( 'NONE', #36287, #7661, #22409 ) ;
#37523=CARTESIAN_POINT ( 'NONE',  ( 454.7528517110262101, 199.9999999999999432, 339.9999999999999432 ) ) ;
#37541=CARTESIAN_POINT ( 'NONE',  ( -919.9999999999993179, 154.9999999999998863, -360.0000000000000000 ) ) ;
#37575=DIRECTION ( 'NONE',  ( -0.000000000000000000, 1.000000000000000000, -0.000000000000000000 ) ) ;
#37585=FACE_OUTER_BOUND ( 'NONE', #22591, .T. ) ;
#37623=CARTESIAN_POINT ( 'NONE',  ( -78.83651009197140525, 230.0000000000000568, -202.7499999999934346 ) ) ;
#37627=EDGE_LOOP ( 'NONE', ( #8759, #20355 ) ) ;
#37688=ORIENTED_EDGE ( 'NONE', *, *, #16791, .F. ) ;
#37699=EDGE_CURVE ( 'NONE', #20516, #43844, #19189, .T. ) ;
#37714=ORIENTED_EDGE ( 'NONE', *, *, #27824, .T. ) ;
#37746=CARTESIAN_POINT ( 'NONE',  ( 928.0249999999991815, 154.9999999999998863, 350.0000000000000000 ) ) ;
#37789=ORIENTED_EDGE ( 'NONE', *, *, #17924, .T. ) ;
#37796=DIRECTION ( 'NONE',  ( 0.000000000000000000, 0.000000000000000000, 1.000000000000000000 ) ) ;
#37801=AXIS2_PLACEMENT_3D ( 'NONE', #26030, #1341, #8506 ) ;
#37826=DIRECTION ( 'NONE',  ( 1.000000000000000000, 0.000000000000000000, 0.000000000000000000 ) ) ;
#37850=EDGE_LOOP ( 'NONE', ( #15000, #18543 ) ) ;
#37942=ORIENTED_EDGE ( 'NONE', *, *, #31178, .T. ) ;
#37965=EDGE_CURVE ( 'NONE', #40984, #23028, #39812, .T. ) ;
#37974=EDGE_CURVE ( 'NONE', #39962, #9635, #25743, .T. ) ;
#38003=VECTOR ( 'NONE', #6521, 1000.000000000000000 ) ;
#38017=DIRECTION ( 'NONE',  ( 1.000000000000000000, 0.000000000000000000, 0.000000000000000000 ) ) ;
#38040=AXIS2_PLACEMENT_3D ( 'NONE', #41215, #34036, #30574 ) ;
#38043=FACE_OUTER_BOUND ( 'NONE', #22784, .T. ) ;
#38045=FACE_OUTER_BOUND ( 'NONE', #31129, .T. ) ;
#38065=PLANE ( 'NONE',  #25444 ) ;
#38080=ORIENTED_EDGE ( 'NONE', *, *, #16833, .F. ) ;
#38163=EDGE_CURVE ( 'NONE', #19824, #1441, #30479, .T. ) ;
#38164=CARTESIAN_POINT ( 'NONE',  ( -919.9999999999993179, 219.9999999999998863, 339.9999999999999432 ) ) ;
#38168=CARTESIAN_POINT ( 'NONE',  ( -959.5497976682736407, 240.0000000000002274, -2132.806278688367456 ) ) ;
#38190=CYLINDRICAL_SURFACE ( 'NONE', #41904, 2.749999999999863665 ) ;
#38202=CARTESIAN_POINT ( 'NONE',  ( -454.7528517110260964, 240.0000000000001421, 350.0000000000000000 ) ) ;
#38207=LINE ( 'NONE', #6330, #15268 ) ;
#38224=CYLINDRICAL_SURFACE ( 'NONE', #9894, 2.749999999999835687 ) ;
#38237=EDGE_CURVE ( 'NONE', #17262, #10523, #19868, .T. ) ;
#38328=ORIENTED_EDGE ( 'NONE', *, *, #6873, .T. ) ;
#38338=CARTESIAN_POINT ( 'NONE',  ( -208.8365100919714052, 260.0000000000001137, -202.7499999999925251 ) ) ;
#38341=AXIS2_PLACEMENT_3D ( 'NONE', #770, #4250, #15087 ) ;
#38424=DIRECTION ( 'NONE',  ( -1.880165489482579047E-16, -1.000000000000000000, 0.000000000000000000 ) ) ;
#38461=FACE_OUTER_BOUND ( 'NONE', #31182, .T. ) ;
#38486=DIRECTION ( 'NONE',  ( 0.000000000000000000, 0.000000000000000000, 1.000000000000000000 ) ) ;
#38491=CARTESIAN_POINT ( 'NONE',  ( 311.1634899080286232, 240.0000000000000000, -199.9999999999963336 ) ) ;
#38506=ADVANCED_FACE ( 'NONE', ( #42254, #10612, #24688, #14313, #35317, #3695, #5635, #29059, #25809, #4355, #39922, #4795, #19959, #22330, #5869 ), #34033, .F. ) ;
#38605=CARTESIAN_POINT ( 'NONE',  ( 911.9749999999993406, 219.9999999999998863, 339.9999999999999432 ) ) ;
#38619=VECTOR ( 'NONE', #14822, 1000.000000000000000 ) ;
#38640=ORIENTED_EDGE ( 'NONE', *, *, #13433, .F. ) ;
#38643=VERTEX_POINT ( 'NONE', #32752 ) ;
#38649=ORIENTED_EDGE ( 'NONE', *, *, #18500, .T. ) ;
#38654=CYLINDRICAL_SURFACE ( 'NONE', #38341, 8.024999999999948841 ) ;
#38659=AXIS2_PLACEMENT_3D ( 'NONE', #31278, #30595, #13283 ) ;
#38662=AXIS2_PLACEMENT_3D ( 'NONE', #2412, #5414, #40999 ) ;
#38727=DIRECTION ( 'NONE',  ( 1.000000000000000000, 0.000000000000000000, 0.000000000000000000 ) ) ;
#38735=DIRECTION ( 'NONE',  ( 0.000000000000000000, 0.000000000000000000, 1.000000000000000000 ) ) ;
#38737=AXIS2_PLACEMENT_3D ( 'NONE', #38164, #34211, #20366 ) ;
#38741=ADVANCED_FACE ( 'NONE', ( #37275 ), #8054, .F. ) ;
#38760=ORIENTED_EDGE ( 'NONE', *, *, #25747, .T. ) ;
#38843=DIRECTION ( 'NONE',  ( -1.000000000000000000, 1.880165489482579047E-16, 0.000000000000000000 ) ) ;
#38902=DIRECTION ( 'NONE',  ( -1.000000000000000000, 0.000000000000000000, 0.000000000000000000 ) ) ;
#38904=ORIENTED_EDGE ( 'NONE', *, *, #40553, .T. ) ;
#38935=DIRECTION ( 'NONE',  ( -1.000000000000000000, 0.000000000000000000, 0.000000000000000000 ) ) ;
#38973=CYLINDRICAL_SURFACE ( 'NONE', #16428, 8.024999999999948841 ) ;
#39003=SHAPE_DEFINITION_REPRESENTATION ( #7477, #18903 ) ;
#39020=DIRECTION ( 'NONE',  ( -1.880165489482579047E-16, -1.000000000000000000, -0.000000000000000000 ) ) ;
#39023=ORIENTED_EDGE ( 'NONE', *, *, #39102, .F. ) ;
#39027=DIRECTION ( 'NONE',  ( -1.880165489482579047E-16, -1.000000000000000000, -0.000000000000000000 ) ) ;
#39054=CARTESIAN_POINT ( 'NONE',  ( 919.9999999999993179, 219.9999999999998863, 350.0000000000000000 ) ) ;
#39102=EDGE_CURVE ( 'NONE', #10345, #1685, #5129, .T. ) ;
#39108=DIRECTION ( 'NONE',  ( -1.000000000000000000, 0.000000000000000000, 0.000000000000000000 ) ) ;
#39132=EDGE_CURVE ( 'NONE', #10075, #12108, #6552, .T. ) ;
#39136=ADVANCED_FACE ( 'NONE', ( #24541 ), #38654, .F. ) ;
#39142=DIRECTION ( 'NONE',  ( -0.000000000000000000, 1.000000000000000000, -0.000000000000000000 ) ) ;
#39158=EDGE_LOOP ( 'NONE', ( #22269, #15542, #25967, #43159, #39379, #139, #16189, #21074, #20398, #16898, #5348, #15737 ) ) ;
#39164=DIRECTION ( 'NONE',  ( 1.000000000000000000, 0.000000000000000000, 0.000000000000000000 ) ) ;
#39194=DIRECTION ( 'NONE',  ( 1.000000000000000000, 0.000000000000000000, 0.000000000000000000 ) ) ;
#39244=EDGE_LOOP ( 'NONE', ( #15979, #25907, #13716, #44543 ) ) ;
#39336=VERTEX_POINT ( 'NONE', #22226 ) ;
#39345=DIRECTION ( 'NONE',  ( -0.000000000000000000, 1.000000000000000000, -0.000000000000000000 ) ) ;
#39379=ORIENTED_EDGE ( 'NONE', *, *, #9206, .T. ) ;
#39387=EDGE_CURVE ( 'NONE', #36831, #5978, #10945, .T. ) ;
#39449=EDGE_LOOP ( 'NONE', ( #32463, #709, #2466, #2612 ) ) ;
#39475=EDGE_CURVE ( 'NONE', #5289, #42219, #39590, .T. ) ;
#39484=LINE ( 'NONE', #21679, #18242 ) ;
#39499=DIRECTION ( 'NONE',  ( -1.880165489482579047E-16, -1.000000000000000000, -0.000000000000000000 ) ) ;
#39501=VECTOR ( 'NONE', #948, 1000.000000000000000 ) ;
#39509=ORIENTED_EDGE ( 'NONE', *, *, #6873, .F. ) ;
#39532=DIRECTION ( 'NONE',  ( -1.880165489482579047E-16, -1.000000000000000000, -0.000000000000000000 ) ) ;
#39553=CIRCLE ( 'NONE', #18869, 2.749999999999919176 ) ;
#39558=FACE_OUTER_BOUND ( 'NONE', #33468, .T. ) ;
#39590=LINE ( 'NONE', #29174, #34444 ) ;
#39638=CIRCLE ( 'NONE', #1270, 2.749999999999863665 ) ;
#39653=DIRECTION ( 'NONE',  ( 0.000000000000000000, 0.000000000000000000, 1.000000000000000000 ) ) ;
#39660=VECTOR ( 'NONE', #29461, 1000.000000000000000 ) ;
#39673=EDGE_CURVE ( 'NONE', #40984, #24071, #40691, .T. ) ;
#39681=CIRCLE ( 'NONE', #23405, 2.749999999999835687 ) ;
#39685=DIRECTION ( 'NONE',  ( -0.000000000000000000, 1.000000000000000000, -0.000000000000000000 ) ) ;
#39688=ORIENTED_EDGE ( 'NONE', *, *, #41073, .F. ) ;
#39693=ADVANCED_FACE ( 'NONE', ( #23357, #43698, #22447, #4682, #29620 ), #8833, .T. ) ;
#39729=LINE ( 'NONE', #8077, #22519 ) ;
#39742=EDGE_CURVE ( 'NONE', #13253, #24672, #19671, .T. ) ;
#39755=PRODUCT_DEFINITION ( 'UNKNOWN', '', #23069, #9939 ) ;
#39786=FACE_OUTER_BOUND ( 'NONE', #28015, .T. ) ;
#39807=ORIENTED_EDGE ( 'NONE', *, *, #14605, .T. ) ;
#39811=EDGE_LOOP ( 'NONE', ( #45468, #25108, #18603, #7005 ) ) ;
#39812=CIRCLE ( 'NONE', #44936, 2.749999999999835687 ) ;
#39820=VERTEX_POINT ( 'NONE', #1653 ) ;
#39901=EDGE_CURVE ( 'NONE', #43290, #42109, #5820, .T. ) ;
#39922=FACE_BOUND ( 'NONE', #3447, .T. ) ;
#39930=DIRECTION ( 'NONE',  ( -0.000000000000000000, 1.000000000000000000, -0.000000000000000000 ) ) ;
#39949=VERTEX_POINT ( 'NONE', #2811 ) ;
#39962=VERTEX_POINT ( 'NONE', #6264 ) ;
#39979=EDGE_CURVE ( 'NONE', #36831, #296, #20579, .T. ) ;
#39998=AXIS2_PLACEMENT_3D ( 'NONE', #41972, #24168, #17937 ) ;
#40086=CARTESIAN_POINT ( 'NONE',  ( 454.7528517110262101, 199.9999999999999432, 350.0000000000000000 ) ) ;
#40118=ORIENTED_EDGE ( 'NONE', *, *, #25210, .T. ) ;
#40137=DIRECTION ( 'NONE',  ( -1.000000000000000000, 0.000000000000000000, 0.000000000000000000 ) ) ;
#40138=CARTESIAN_POINT ( 'NONE',  ( 959.5497976682736407, 120.6654763175833693, -2132.806278688367456 ) ) ;
#40146=VECTOR ( 'NONE', #16715, 1000.000000000000000 ) ;
#40169=EDGE_LOOP ( 'NONE', ( #30232, #3261 ) ) ;
#40176=ORIENTED_EDGE ( 'NONE', *, *, #27775, .F. ) ;
#40193=CARTESIAN_POINT ( 'NONE',  ( 928.0249999999991815, 219.9999999999998863, -360.0000000000000000 ) ) ;
#40215=VECTOR ( 'NONE', #17308, 1000.000000000000000 ) ;
#40218=CIRCLE ( 'NONE', #38737, 8.024999999999948841 ) ;
#40260=LINE ( 'NONE', #36777, #42517 ) ;
#40295=VECTOR ( 'NONE', #29245, 1000.000000000000000 ) ;
#40349=LINE ( 'NONE', #33620, #9950 ) ;
#40351=DIRECTION ( 'NONE',  ( -0.000000000000000000, -0.000000000000000000, -1.000000000000000000 ) ) ;
#40410=ORIENTED_EDGE ( 'NONE', *, *, #4111, .F. ) ;
#40448=ADVANCED_FACE ( 'NONE', ( #42522 ), #7889, .F. ) ;
#40475=ORIENTED_EDGE ( 'NONE', *, *, #17049, .F. ) ;
#40482=CARTESIAN_POINT ( 'NONE',  ( -911.9749999999993406, 154.9999999999998863, 339.9999999999999432 ) ) ;
#40496=EDGE_CURVE ( 'NONE', #5848, #15202, #10887, .T. ) ;
#40500=FACE_BOUND ( 'NONE', #42856, .T. ) ;
#40502=LINE ( 'NONE', #12539, #31358 ) ;
#40509=ORIENTED_EDGE ( 'NONE', *, *, #35022, .F. ) ;
#40553=EDGE_CURVE ( 'NONE', #7179, #13769, #40831, .T. ) ;
#40563=CARTESIAN_POINT ( 'NONE',  ( 454.7528517110262101, 229.9999999999999432, -2132.806278688367456 ) ) ;
#40568=EDGE_CURVE ( 'NONE', #32683, #7811, #36267, .T. ) ;
#40580=ORIENTED_EDGE ( 'NONE', *, *, #17924, .F. ) ;
#40608=ORIENTED_EDGE ( 'NONE', *, *, #1581, .F. ) ;
#40615=ORIENTED_EDGE ( 'NONE', *, *, #30034, .F. ) ;
#40641=DIRECTION ( 'NONE',  ( 0.000000000000000000, 0.000000000000000000, 1.000000000000000000 ) ) ;
#40644=ORIENTED_EDGE ( 'NONE', *, *, #4374, .T. ) ;
#40673=CARTESIAN_POINT ( 'NONE',  ( -598.8365100919716042, 260.0000000000001705, -202.7499999999898250 ) ) ;
#40691=LINE ( 'NONE', #44380, #20433 ) ;
#40692=CARTESIAN_POINT ( 'NONE',  ( -468.8365100919714337, 230.0000000000001421, -199.9999999999908766 ) ) ;
#40706=CARTESIAN_POINT ( 'NONE',  ( 521.6730038022808458, 229.9999999999999432, -122.7905160835442615 ) ) ;
#40712=CARTESIAN_POINT ( 'NONE',  ( 441.1634899080286232, 229.9999999999999716, -197.2499999999973852 ) ) ;
#40729=( LENGTH_UNIT ( ) NAMED_UNIT ( * ) SI_UNIT ( .MILLI., .METRE. ) );
#40733=AXIS2_PLACEMENT_3D ( 'NONE', #43756, #22748, #36843 ) ;
#40817=ADVANCED_FACE ( 'NONE', ( #8322 ), #36724, .F. ) ;
#40820=VERTEX_POINT ( 'NONE', #8781 ) ;
#40823=DIRECTION ( 'NONE',  ( -1.880165489482579047E-16, -1.000000000000000000, -0.000000000000000000 ) ) ;
#40828=VECTOR ( 'NONE', #654, 1000.000000000000000 ) ;
#40831=CIRCLE ( 'NONE', #34925, 2.749999999999919176 ) ;
#40837=ORIENTED_EDGE ( 'NONE', *, *, #33769, .F. ) ;
#40846=DIRECTION ( 'NONE',  ( 1.000000000000000000, 0.000000000000000000, 0.000000000000000000 ) ) ;
#40886=DIRECTION ( 'NONE',  ( 1.000000000000000000, 0.000000000000000000, 0.000000000000000000 ) ) ;
#40927=VECTOR ( 'NONE', #31396, 1000.000000000000000 ) ;
#40964=DIRECTION ( 'NONE',  ( 1.000000000000000000, 0.000000000000000000, 0.000000000000000000 ) ) ;
#40984=VERTEX_POINT ( 'NONE', #37623 ) ;
#40991=DIRECTION ( 'NONE',  ( -0.000000000000000000, 1.000000000000000000, -0.000000000000000000 ) ) ;
#40999=DIRECTION ( 'NONE',  ( 1.000000000000000000, 0.000000000000000000, 0.000000000000000000 ) ) ;
#41013=CARTESIAN_POINT ( 'NONE',  ( 919.9999999999993179, 154.9999999999998863, 350.0000000000000000 ) ) ;
#41016=CIRCLE ( 'NONE', #36566, 2.749999999999842792 ) ;
#41073=EDGE_CURVE ( 'NONE', #1769, #44135, #5760, .T. ) ;
#41081=VECTOR ( 'NONE', #2334, 1000.000000000000000 ) ;
#41103=EDGE_CURVE ( 'NONE', #10523, #13769, #30705, .T. ) ;
#41105=AXIS2_PLACEMENT_3D ( 'NONE', #34625, #15928, #30011 ) ;
#41150=ORIENTED_EDGE ( 'NONE', *, *, #1475, .T. ) ;
#41159=ORIENTED_EDGE ( 'NONE', *, *, #42189, .F. ) ;
#41180=LINE ( 'NONE', #9755, #29873 ) ;
#41187=FACE_OUTER_BOUND ( 'NONE', #22314, .T. ) ;
#41190=VERTEX_POINT ( 'NONE', #20746 ) ;
#41211=CARTESIAN_POINT ( 'NONE',  ( -338.8365100919713200, 260.0000000000001137, -197.2499999999919282 ) ) ;
#41215=CARTESIAN_POINT ( 'NONE',  ( -919.9999999999993179, 154.9999999999998863, 339.9999999999999432 ) ) ;
#41300=CARTESIAN_POINT ( 'NONE',  ( -521.6730038022808458, 240.0000000000001705, -122.7905160835438068 ) ) ;
#41330=EDGE_CURVE ( 'NONE', #44890, #15534, #4697, .T. ) ;
#41350=CARTESIAN_POINT ( 'NONE',  ( -78.83651009197140525, 230.0000000000000568, -199.9999999999936051 ) ) ;
#41414=ORIENTED_EDGE ( 'NONE', *, *, #33769, .T. ) ;
#41439=LINE ( 'NONE', #43862, #3455 ) ;
#41455=CARTESIAN_POINT ( 'NONE',  ( -208.8365100919714052, 260.0000000000001137, -199.9999999999926956 ) ) ;
#41475=CARTESIAN_POINT ( 'NONE',  ( 51.16348990802859475, 240.0000000000000568, -197.2499999999946851 ) ) ;
#41495=AXIS2_PLACEMENT_3D ( 'NONE', #2235, #41504, #6158 ) ;
#41504=DIRECTION ( 'NONE',  ( -1.880165489482579047E-16, -1.000000000000000000, -0.000000000000000000 ) ) ;
#41522=FACE_BOUND ( 'NONE', #45356, .T. ) ;
#41536=ORIENTED_EDGE ( 'NONE', *, *, #7420, .F. ) ;
#41566=CARTESIAN_POINT ( 'NONE',  ( 831.1634899080286232, 259.9999999999998863, -197.2500000000000853 ) ) ;
#41569=( GEOMETRIC_REPRESENTATION_CONTEXT ( 3 ) GLOBAL_UNCERTAINTY_ASSIGNED_CONTEXT ( ( #6702 ) ) GLOBAL_UNIT_ASSIGNED_CONTEXT ( ( #15190, #853, #21878 ) ) REPRESENTATION_CONTEXT ( 'NONE', 'WORKASPACE' ) );
#41581=ORIENTED_EDGE ( 'NONE', *, *, #3591, .F. ) ;
#41588=VECTOR ( 'NONE', #38735, 1000.000000000000000 ) ;
#41633=DIRECTION ( 'NONE',  ( 0.000000000000000000, 0.000000000000000000, 1.000000000000000000 ) ) ;
#41634=AXIS2_PLACEMENT_3D ( 'NONE', #30440, #2263, #40846 ) ;
#41653=ADVANCED_FACE ( 'NONE', ( #22128 ), #1766, .F. ) ;
#41675=CARTESIAN_POINT ( 'NONE',  ( 949.5497976682736407, 120.6654763175833693, -2132.806278688367456 ) ) ;
#41682=VECTOR ( 'NONE', #33848, 1000.000000000000000 ) ;
#41739=CYLINDRICAL_SURFACE ( 'NONE', #17873, 2.749999999999863665 ) ;
#41787=ORIENTED_EDGE ( 'NONE', *, *, #30289, .T. ) ;
#41874=CARTESIAN_POINT ( 'NONE',  ( 311.1634899080286232, 240.0000000000000000, -197.2499999999964473 ) ) ;
#41897=VERTEX_POINT ( 'NONE', #29965 ) ;
#41904=AXIS2_PLACEMENT_3D ( 'NONE', #23613, #6762, #2846 ) ;
#41924=EDGE_CURVE ( 'NONE', #41190, #21010, #43596, .T. ) ;
#41944=EDGE_CURVE ( 'NONE', #19824, #14734, #12417, .T. ) ;
#41951=ORIENTED_EDGE ( 'NONE', *, *, #23016, .T. ) ;
#41967=CARTESIAN_POINT ( 'NONE',  ( -454.7528517110260964, 200.0000000000001137, 350.0000000000000000 ) ) ;
#41972=CARTESIAN_POINT ( 'NONE',  ( -919.9999999999993179, 154.9999999999998863, -360.0000000000000000 ) ) ;
#41978=CARTESIAN_POINT ( 'NONE',  ( 521.6730038022808458, 229.9999999999999432, -2132.806278688367456 ) ) ;
#41979=AXIS2_PLACEMENT_3D ( 'NONE', #10908, #24976, #3519 ) ;
#42033=DIRECTION ( 'NONE',  ( -1.880165489482579047E-16, -1.000000000000000000, -0.000000000000000000 ) ) ;
#42079=FACE_OUTER_BOUND ( 'NONE', #2545, .T. ) ;
#42099=ORIENTED_EDGE ( 'NONE', *, *, #5239, .F. ) ;
#42109=VERTEX_POINT ( 'NONE', #27407 ) ;
#42126=CARTESIAN_POINT ( 'NONE',  ( 911.9749999999993406, 154.9999999999998863, 350.0000000000000000 ) ) ;
#42170=CARTESIAN_POINT ( 'NONE',  ( 949.5497976682736407, 120.6654763175833693, 339.9999999999999432 ) ) ;
#42173=EDGE_CURVE ( 'NONE', #16933, #24181, #15673, .T. ) ;
#42189=EDGE_CURVE ( 'NONE', #33196, #19590, #44280, .T. ) ;
#42193=ADVANCED_FACE ( 'NONE', ( #24169 ), #30880, .F. ) ;
#42219=VERTEX_POINT ( 'NONE', #30651 ) ;
#42229=CARTESIAN_POINT ( 'NONE',  ( 959.5497976682736407, 239.9999999999998863, 350.0000000000000000 ) ) ;
#42249=AXIS2_PLACEMENT_3D ( 'NONE', #12135, #1713, #43540 ) ;
#42254=FACE_BOUND ( 'NONE', #16958, .T. ) ;
#42262=ADVANCED_FACE ( 'NONE', ( #20246 ), #2009, .F. ) ;
#42343=CIRCLE ( 'NONE', #38662, 2.749999999999919176 ) ;
#42345=DIRECTION ( 'NONE',  ( 0.000000000000000000, 0.000000000000000000, -1.000000000000000000 ) ) ;
#42368=DIRECTION ( 'NONE',  ( 1.000000000000000000, 0.000000000000000000, 0.000000000000000000 ) ) ;
#42375=CIRCLE ( 'NONE', #2540, 2.749999999999863665 ) ;
#42389=CIRCLE ( 'NONE', #26878, 8.024999999999948841 ) ;
#42422=DIRECTION ( 'NONE',  ( -0.000000000000000000, 1.000000000000000000, -0.000000000000000000 ) ) ;
#42428=DIRECTION ( 'NONE',  ( 1.000000000000000000, 0.000000000000000000, 0.000000000000000000 ) ) ;
#42451=CIRCLE ( 'NONE', #29921, 2.749999999999919176 ) ;
#42492=EDGE_CURVE ( 'NONE', #23058, #32406, #5367, .T. ) ;
#42498=ORIENTED_EDGE ( 'NONE', *, *, #45245, .F. ) ;
#42517=VECTOR ( 'NONE', #22446, 1000.000000000000000 ) ;
#42522=FACE_OUTER_BOUND ( 'NONE', #26179, .T. ) ;
#42536=AXIS2_PLACEMENT_3D ( 'NONE', #24163, #23920, #13326 ) ;
#42584=DIRECTION ( 'NONE',  ( -0.000000000000000000, -0.000000000000000000, -1.000000000000000000 ) ) ;
#42588=CARTESIAN_POINT ( 'NONE',  ( 831.1634899080286232, 239.9999999999999147, -199.9999999999999432 ) ) ;
#42609=CARTESIAN_POINT ( 'NONE',  ( -598.8365100919716042, 260.0000000000001705, -197.2499999999901092 ) ) ;
#42648=LINE ( 'NONE', #31566, #37266 ) ;
#42651=DIRECTION ( 'NONE',  ( 1.000000000000000000, 0.000000000000000000, 0.000000000000000000 ) ) ;
#42692=LINE ( 'NONE', #22124, #29992 ) ;
#42693=CARTESIAN_POINT ( 'NONE',  ( -338.8365100919713200, 240.0000000000001421, -202.7499999999916724 ) ) ;
#42732=EDGE_CURVE ( 'NONE', #30067, #39949, #14993, .T. ) ;
#42746=ORIENTED_EDGE ( 'NONE', *, *, #23016, .F. ) ;
#42762=ADVANCED_FACE ( 'NONE', ( #7090 ), #38973, .F. ) ;
#42767=CARTESIAN_POINT ( 'NONE',  ( 879.9999999999990905, 479.9999999999998863, -210.0000000000000000 ) ) ;
#42777=ORIENTED_EDGE ( 'NONE', *, *, #43893, .F. ) ;
#42784=EDGE_LOOP ( 'NONE', ( #34999, #12158, #25397, #25960 ) ) ;
#42786=EDGE_CURVE ( 'NONE', #32578, #9428, #43719, .T. ) ;
#42802=LINE ( 'NONE', #21779, #18887 ) ;
#42856=EDGE_LOOP ( 'NONE', ( #34553, #39023 ) ) ;
#42927=AXIS2_PLACEMENT_3D ( 'NONE', #20029, #20494, #34106 ) ;
#42970=VERTEX_POINT ( 'NONE', #40086 ) ;
#42992=DIRECTION ( 'NONE',  ( 0.000000000000000000, 0.000000000000000000, -1.000000000000000000 ) ) ;
#43025=CARTESIAN_POINT ( 'NONE',  ( 919.9999999999993179, 219.9999999999998863, 339.9999999999999432 ) ) ;
#43029=ORIENTED_EDGE ( 'NONE', *, *, #40568, .F. ) ;
#43060=ORIENTED_EDGE ( 'NONE', *, *, #24640, .T. ) ;
#43072=ORIENTED_EDGE ( 'NONE', *, *, #8870, .F. ) ;
#43073=CIRCLE ( 'NONE', #15766, 2.749999999999835687 ) ;
#43090=VECTOR ( 'NONE', #13732, 1000.000000000000000 ) ;
#43091=CARTESIAN_POINT ( 'NONE',  ( 51.16348990802859475, 260.0000000000000568, -199.9999999999945146 ) ) ;
#43092=CARTESIAN_POINT ( 'NONE',  ( -338.8365100919713200, 230.0000000000001137, -197.2499999999919282 ) ) ;
#43148=DIRECTION ( 'NONE',  ( 1.000000000000000000, 0.000000000000000000, 0.000000000000000000 ) ) ;
#43155=CARTESIAN_POINT ( 'NONE',  ( 919.9999999999993179, 154.9999999999998863, 339.9999999999999432 ) ) ;
#43159=ORIENTED_EDGE ( 'NONE', *, *, #41073, .T. ) ;
#43172=FACE_OUTER_BOUND ( 'NONE', #25131, .T. ) ;
#43188=VECTOR ( 'NONE', #40351, 1000.000000000000000 ) ;
#43243=ORIENTED_EDGE ( 'NONE', *, *, #45621, .F. ) ;
#43260=EDGE_LOOP ( 'NONE', ( #23035, #40475 ) ) ;
#43263=DIRECTION ( 'NONE',  ( 1.000000000000000000, 0.000000000000000000, 0.000000000000000000 ) ) ;
#43290=VERTEX_POINT ( 'NONE', #37523 ) ;
#43291=AXIS2_PLACEMENT_3D ( 'NONE', #29727, #44275, #12861 ) ;
#43322=DIRECTION ( 'NONE',  ( 0.000000000000000000, 0.000000000000000000, 1.000000000000000000 ) ) ;
#43349=ORIENTED_EDGE ( 'NONE', *, *, #8252, .F. ) ;
#43363=ORIENTED_EDGE ( 'NONE', *, *, #16308, .F. ) ;
#43444=VECTOR ( 'NONE', #29136, 1000.000000000000000 ) ;
#43487=APPLICATION_CONTEXT ( 'automotive_design' ) ;
#43511=CARTESIAN_POINT ( 'NONE',  ( 441.1634899080286232, 229.9999999999999716, -202.7499999999971010 ) ) ;
#43520=ORIENTED_EDGE ( 'NONE', *, *, #21050, .F. ) ;
#43540=DIRECTION ( 'NONE',  ( 1.000000000000000000, 0.000000000000000000, 0.000000000000000000 ) ) ;
#43596=LINE ( 'NONE', #880, #17892 ) ;
#43619=EDGE_CURVE ( 'NONE', #338, #44890, #32370, .T. ) ;
#43638=CIRCLE ( 'NONE', #6013, 8.024999999999948841 ) ;
#43647=DIRECTION ( 'NONE',  ( -0.000000000000000000, 1.000000000000000000, -0.000000000000000000 ) ) ;
#43698=FACE_BOUND ( 'NONE', #18137, .T. ) ;
#43708=CARTESIAN_POINT ( 'NONE',  ( 831.1634899080286232, 239.9999999999999147, -197.2500000000000853 ) ) ;
#43719=CIRCLE ( 'NONE', #42249, 8.024999999999948841 ) ;
#43744=VERTEX_POINT ( 'NONE', #3889 ) ;
#43756=CARTESIAN_POINT ( 'NONE',  ( -338.8365100919713200, 240.0000000000001421, -199.9999999999917861 ) ) ;
#43768=DIRECTION ( 'NONE',  ( -0.000000000000000000, -0.000000000000000000, 1.000000000000000000 ) ) ;
#43788=EDGE_CURVE ( 'NONE', #13142, #39820, #10825, .T. ) ;
#43794=CIRCLE ( 'NONE', #27585, 2.749999999999863665 ) ;
#43810=EDGE_CURVE ( 'NONE', #296, #14734, #24660, .T. ) ;
#43817=EDGE_CURVE ( 'NONE', #8116, #11158, #34919, .T. ) ;
#43820=ORIENTED_EDGE ( 'NONE', *, *, #1581, .T. ) ;
#43844=VERTEX_POINT ( 'NONE', #424 ) ;
#43847=CIRCLE ( 'NONE', #23932, 2.749999999999842792 ) ;
#43854=ORIENTED_EDGE ( 'NONE', *, *, #37699, .F. ) ;
#43860=EDGE_CURVE ( 'NONE', #20005, #19031, #21212, .T. ) ;
#43862=CARTESIAN_POINT ( 'NONE',  ( -928.0249999999991815, 219.9999999999998863, -360.0000000000000000 ) ) ;
#43886=DIRECTION ( 'NONE',  ( 0.000000000000000000, 0.000000000000000000, 1.000000000000000000 ) ) ;
#43893=EDGE_CURVE ( 'NONE', #40820, #15260, #22351, .T. ) ;
#43926=CARTESIAN_POINT ( 'NONE',  ( 0.000000000000000000, 0.000000000000000000, 339.9999999999999432 ) ) ;
#43940=DIRECTION ( 'NONE',  ( 1.000000000000000000, 0.000000000000000000, 0.000000000000000000 ) ) ;
#44029=VECTOR ( 'NONE', #16434, 1000.000000000000000 ) ;
#44095=ORIENTED_EDGE ( 'NONE', *, *, #30571, .F. ) ;
#44135=VERTEX_POINT ( 'NONE', #12642 ) ;
#44175=DIRECTION ( 'NONE',  ( -0.000000000000000000, 1.000000000000000000, -0.000000000000000000 ) ) ;
#44179=CARTESIAN_POINT ( 'NONE',  ( 919.9999999999993179, 219.9999999999998863, 350.0000000000000000 ) ) ;
#44263=ORIENTED_EDGE ( 'NONE', *, *, #4417, .T. ) ;
#44275=DIRECTION ( 'NONE',  ( -1.880165489482579047E-16, -1.000000000000000000, -0.000000000000000000 ) ) ;
#44280=LINE ( 'NONE', #2464, #33371 ) ;
#44330=VERTEX_POINT ( 'NONE', #24615 ) ;
#44380=CARTESIAN_POINT ( 'NONE',  ( -78.83651009197140525, 260.0000000000000568, -202.7499999999934346 ) ) ;
#44382=ORIENTED_EDGE ( 'NONE', *, *, #402, .T. ) ;
#44442=EDGE_CURVE ( 'NONE', #44330, #21264, #43073, .T. ) ;
#44452=DIRECTION ( 'NONE',  ( -1.000000000000000000, 0.000000000000000000, -0.000000000000000000 ) ) ;
#44469=CARTESIAN_POINT ( 'NONE',  ( -338.8365100919713200, 240.0000000000001421, -197.2499999999919282 ) ) ;
#44480=EDGE_CURVE ( 'NONE', #2099, #1769, #17495, .T. ) ;
#44488=VERTEX_POINT ( 'NONE', #10098 ) ;
#44503=ADVANCED_FACE ( 'NONE', ( #21176 ), #6628, .F. ) ;
#44506=DIRECTION ( 'NONE',  ( 0.000000000000000000, 0.000000000000000000, 1.000000000000000000 ) ) ;
#44543=ORIENTED_EDGE ( 'NONE', *, *, #4374, .F. ) ;
#44574=VECTOR ( 'NONE', #27366, 1000.000000000000000 ) ;
#44639=EDGE_CURVE ( 'NONE', #39336, #33570, #20934, .T. ) ;
#44677=LINE ( 'NONE', #5638, #12214 ) ;
#44706=VECTOR ( 'NONE', #33448, 1000.000000000000000 ) ;
#44723=ADVANCED_FACE ( 'NONE', ( #8013 ), #32947, .F. ) ;
#44726=ORIENTED_EDGE ( 'NONE', *, *, #8298, .F. ) ;
#44748=DIRECTION ( 'NONE',  ( -0.000000000000000000, 1.000000000000000000, -0.000000000000000000 ) ) ;
#44771=VERTEX_POINT ( 'NONE', #29017 ) ;
#44783=CIRCLE ( 'NONE', #43291, 2.749999999999919176 ) ;
#44845=VERTEX_POINT ( 'NONE', #7327 ) ;
#44878=DIRECTION ( 'NONE',  ( 0.000000000000000000, -1.000000000000000000, 0.000000000000000000 ) ) ;
#44890=VERTEX_POINT ( 'NONE', #4314 ) ;
#44936=AXIS2_PLACEMENT_3D ( 'NONE', #41350, #37180, #40886 ) ;
#44947=DIRECTION ( 'NONE',  ( 0.000000000000000000, 0.000000000000000000, 1.000000000000000000 ) ) ;
#45130=DIRECTION ( 'NONE',  ( 1.000000000000000000, 0.000000000000000000, 0.000000000000000000 ) ) ;
#45195=CARTESIAN_POINT ( 'NONE',  ( 831.1634899080286232, 259.9999999999998863, -199.9999999999999432 ) ) ;
#45200=CARTESIAN_POINT ( 'NONE',  ( -208.8365100919714052, 240.0000000000001137, -199.9999999999926956 ) ) ;
#45245=EDGE_CURVE ( 'NONE', #24787, #296, #11911, .T. ) ;
#45285=VECTOR ( 'NONE', #26892, 1000.000000000000000 ) ;
#45286=ORIENTED_EDGE ( 'NONE', *, *, #4645, .F. ) ;
#45319=DIRECTION ( 'NONE',  ( 1.000000000000000000, 0.000000000000000000, 0.000000000000000000 ) ) ;
#45335=CIRCLE ( 'NONE', #1084, 2.749999999999863665 ) ;
#45339=ORIENTED_EDGE ( 'NONE', *, *, #25811, .T. ) ;
#45356=EDGE_LOOP ( 'NONE', ( #20837, #18645 ) ) ;
#45376=CIRCLE ( 'NONE', #2557, 2.749999999999919176 ) ;
#45382=DIRECTION ( 'NONE',  ( 0.000000000000000000, 0.000000000000000000, 1.000000000000000000 ) ) ;
#45435=CYLINDRICAL_SURFACE ( 'NONE', #39998, 8.024999999999948841 ) ;
#45468=ORIENTED_EDGE ( 'NONE', *, *, #43860, .F. ) ;
#45490=ADVANCED_FACE ( 'NONE', ( #6347 ), #16749, .F. ) ;
#45526=ORIENTED_EDGE ( 'NONE', *, *, #25849, .F. ) ;
#45541=CARTESIAN_POINT ( 'NONE',  ( 959.5497976682736407, 239.9999999999998863, 350.0000000000000000 ) ) ;
#45562=ADVANCED_FACE ( 'NONE', ( #34524 ), #38224, .F. ) ;
#45583=LINE ( 'NONE', #36087, #593 ) ;
#45596=EDGE_CURVE ( 'NONE', #21264, #44330, #35717, .T. ) ;
#45621=EDGE_CURVE ( 'NONE', #33196, #20005, #20964, .T. ) ;
#45627=ADVANCED_FACE ( 'NONE', ( #26633 ), #27109, .F. ) ;
#45635=VERTEX_POINT ( 'NONE', #33574 ) ;
#45656=FACE_OUTER_BOUND ( 'NONE', #34933, .T. ) ;
#45666=DIRECTION ( 'NONE',  ( 1.000000000000000000, -1.880165489482579047E-16, 0.000000000000000000 ) ) ;
#45675=EDGE_CURVE ( 'NONE', #5978, #43844, #37030, .T. ) ;
#45738=COLOUR_RGB('Dark Blue',0.08,0.2,0.34);
#45739=FILL_AREA_STYLE_COLOUR('',#45738);
#45740=FILL_AREA_STYLE('',(#45739));
#45741=SURFACE_STYLE_FILL_AREA(#45740);
#45742=SURFACE_SIDE_STYLE('',(#45741));
#45743=SURFACE_STYLE_USAGE(.BOTH.,#45742);
#45744=PRESENTATION_STYLE_ASSIGNMENT((#45743));
ENDSEC;
END-ISO-10303-21;
